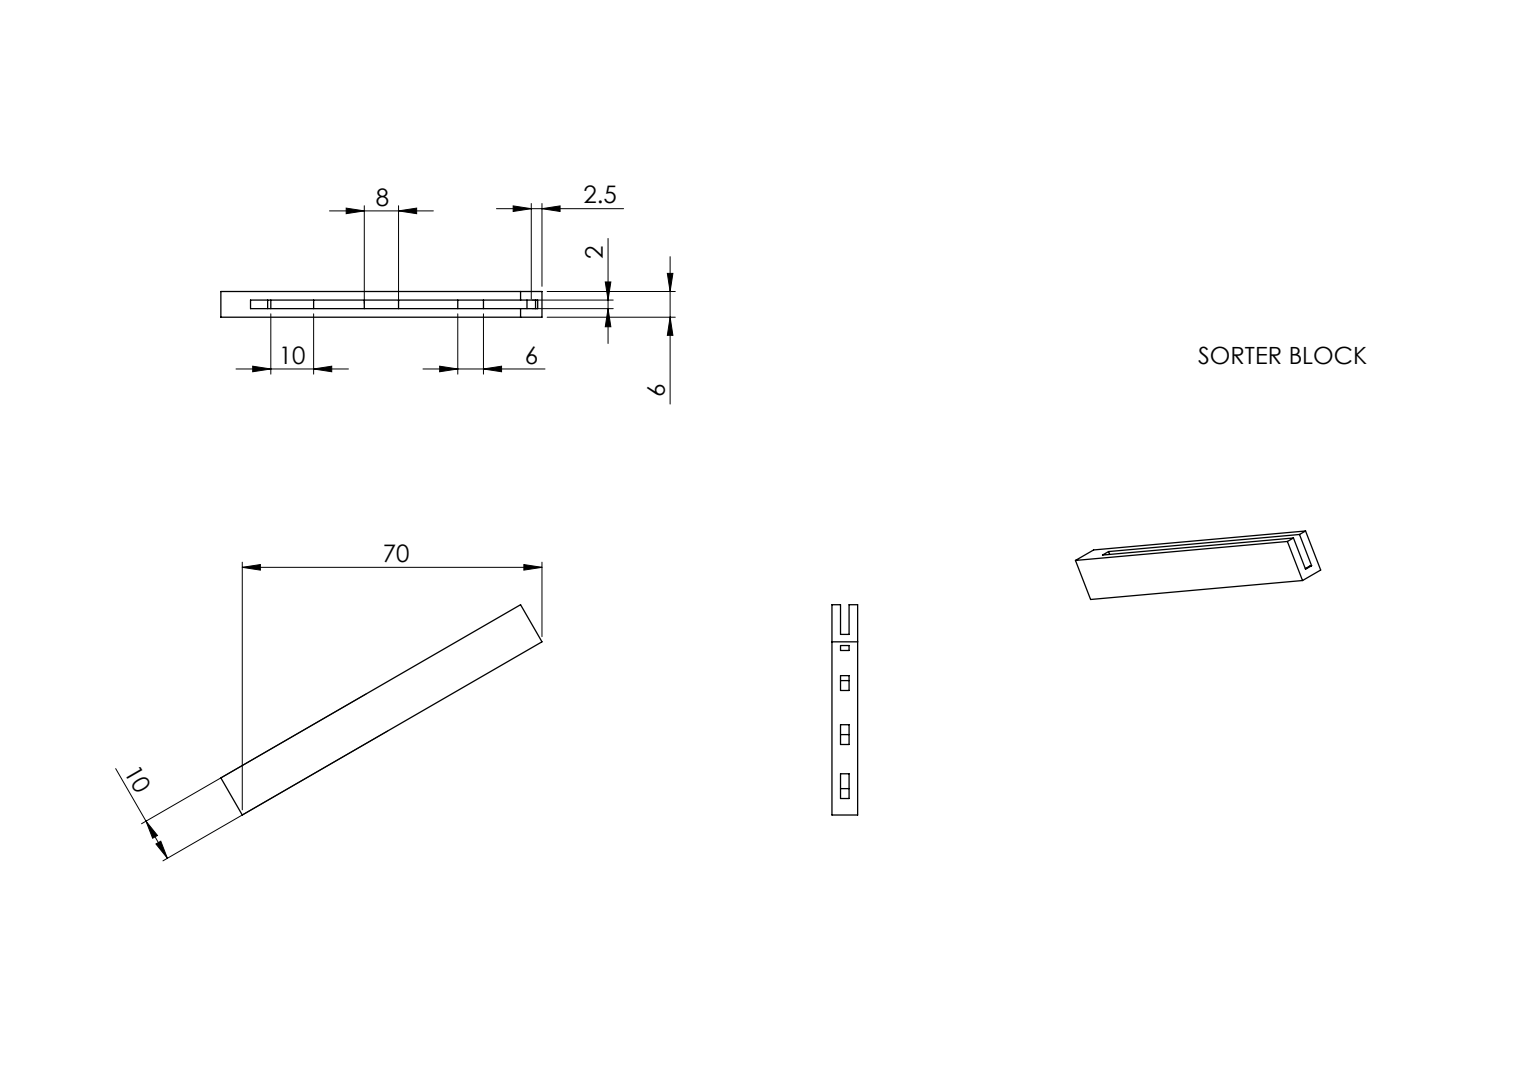
ISO-10303-21;
HEADER;
FILE_DESCRIPTION (('STEP AP214'),
    '1' );
FILE_NAME ('sorter block.step',
    '2026-10-26T05:17:54',
    ( '' ),
    ( '' ),
    'SwSTEP 2.0',
    'SolidWorks 2026',
    '' );
FILE_SCHEMA (( 'AUTOMOTIVE_DESIGN' ));
ENDSEC;

DATA;
#41=VERTEX_POINT ( 'NONE', #12875 ) ;
#78=PLANE ( 'NONE',  #12219 ) ;
#80=FACE_BOUND ( 'NONE', #12190, .T. ) ;
#96=FACE_OUTER_BOUND ( 'NONE', #3585, .T. ) ;
#117=CARTESIAN_POINT ( 'NONE',  ( -43.33333333333332860, 79.07477288111861924, -1.000000000000001110 ) ) ;
#136=EDGE_CURVE ( 'NONE', #12578, #3097, #7900, .T. ) ;
#159=LINE ( 'NONE', #2018, #4188 ) ;
#160=ORIENTED_EDGE ( 'NONE', *, *, #4406, .F. ) ;
#164=ORIENTED_EDGE ( 'NONE', *, *, #8938, .T. ) ;
#180=CARTESIAN_POINT ( 'NONE',  ( -56.80384757729341771, 34.46410161513777837, 0.000000000000000000 ) ) ;
#182=CARTESIAN_POINT ( 'NONE',  ( -60.38397459621558738, 30.66506350946110260, 0.000000000000000000 ) ) ;
#184=EDGE_CURVE ( 'NONE', #4807, #7972, #8814, .T. ) ;
#195=FACE_OUTER_BOUND ( 'NONE', #1919, .T. ) ;
#202=DIRECTION ( 'NONE',  ( -0.5000000000000042188, 0.8660254037844362651, 0.000000000000000000 ) ) ;
#240=ORIENTED_EDGE ( 'NONE', *, *, #10021, .T. ) ;
#255=VERTEX_POINT ( 'NONE', #12080 ) ;
#258=( GEOMETRIC_REPRESENTATION_CONTEXT ( 3 ) GLOBAL_UNCERTAINTY_ASSIGNED_CONTEXT ( ( #6606 ) ) GLOBAL_UNIT_ASSIGNED_CONTEXT ( ( #8219, #3259, #10305 ) ) REPRESENTATION_CONTEXT ( 'NONE', 'WORKASPACE' ) );
#263=AXIS2_PLACEMENT_3D ( 'NONE', #117, #3851, #2872 ) ;
#269=FACE_OUTER_BOUND ( 'NONE', #11895, .T. ) ;
#271=EDGE_CURVE ( 'NONE', #3833, #3097, #6317, .T. ) ;
#306=VECTOR ( 'NONE', #308, 1000.000000000000114 ) ;
#308=DIRECTION ( 'NONE',  ( 0.8660254037844361541, 0.5000000000000042188, 0.000000000000000000 ) ) ;
#315=ORIENTED_EDGE ( 'NONE', *, *, #7224, .T. ) ;
#329=DIRECTION ( 'NONE',  ( -0.8660254037844360431, -0.5000000000000045519, 0.000000000000000000 ) ) ;
#367=VECTOR ( 'NONE', #8627, 1000.000000000000114 ) ;
#377=CYLINDRICAL_SURFACE ( 'NONE', #4983, 1.500000000000000222 ) ;
#384=AXIS2_PLACEMENT_3D ( 'NONE', #10742, #1980, #7866 ) ;
#388=EDGE_CURVE ( 'NONE', #12930, #2334, #4689, .T. ) ;
#405=CARTESIAN_POINT ( 'NONE',  ( 37.99038105676688559, 21.93375672974103452, 1.000000000000000000 ) ) ;
#418=ORIENTED_EDGE ( 'NONE', *, *, #1473, .F. ) ;
#443=VERTEX_POINT ( 'NONE', #483 ) ;
#474=DIRECTION ( 'NONE',  ( -0.8660254037844360431, -0.5000000000000047740, -0.000000000000000000 ) ) ;
#477=CARTESIAN_POINT ( 'NONE',  ( -28.99038105676692112, 50.21281292110204930, -1.000000000000000000 ) ) ;
#481=CARTESIAN_POINT ( 'NONE',  ( 8.999999999999989342, 72.14656965084313356, -1.000000000000000000 ) ) ;
#483=CARTESIAN_POINT ( 'NONE',  ( 4.999999999999962697, 79.07477288111861924, 3.000000000000000000 ) ) ;
#484=ORIENTED_EDGE ( 'NONE', *, *, #7097, .F. ) ;
#486=DIRECTION ( 'NONE',  ( 4.336808689942017243E-16, 2.503857664561960972E-16, -1.000000000000000000 ) ) ;
#492=ORIENTED_EDGE ( 'NONE', *, *, #5266, .F. ) ;
#500=EDGE_CURVE ( 'NONE', #6408, #3143, #4030, .T. ) ;
#501=ORIENTED_EDGE ( 'NONE', *, *, #9357, .T. ) ;
#526=ORIENTED_EDGE ( 'NONE', *, *, #10407, .T. ) ;
#541=DIRECTION ( 'NONE',  ( 0.000000000000000000, 0.000000000000000000, 1.000000000000000000 ) ) ;
#568=ORIENTED_EDGE ( 'NONE', *, *, #10862, .T. ) ;
#570=CARTESIAN_POINT ( 'NONE',  ( 8.499999999999998224, 79.07477288111861924, 1.000000000000000000 ) ) ;
#576=ORIENTED_EDGE ( 'NONE', *, *, #12211, .T. ) ;
#606=FACE_OUTER_BOUND ( 'NONE', #6514, .T. ) ;
#625=DIRECTION ( 'NONE',  ( -0.8746197064978278313, 0.4848096214037562746, 1.049727191973305270E-16 ) ) ;
#645=VECTOR ( 'NONE', #10208, 1000.000000000000227 ) ;
#667=CARTESIAN_POINT ( 'NONE',  ( -54.07179676972453564, 35.73205080756890339, -1.000000000000000000 ) ) ;
#671=DIRECTION ( 'NONE',  ( 0.8660254037844361541, 0.5000000000000042188, 0.000000000000000000 ) ) ;
#676=ORIENTED_EDGE ( 'NONE', *, *, #11289, .T. ) ;
#685=DIRECTION ( 'NONE',  ( -0.8660254037844361541, -0.5000000000000042188, 9.389466242107218061E-17 ) ) ;
#690=VECTOR ( 'NONE', #8750, 1000.000000000000114 ) ;
#695=LINE ( 'NONE', #11320, #4590 ) ;
#724=ORIENTED_EDGE ( 'NONE', *, *, #4951, .F. ) ;
#728=DIRECTION ( 'NONE',  ( 0.000000000000000000, -1.000000000000000000, 0.000000000000000000 ) ) ;
#778=VECTOR ( 'NONE', #11676, 1000.000000000000000 ) ;
#803=CIRCLE ( 'NONE', #8129, 1.500000000000003331 ) ;
#820=PLANE ( 'NONE',  #10704 ) ;
#878=ORIENTED_EDGE ( 'NONE', *, *, #10870, .F. ) ;
#896=ORIENTED_EDGE ( 'NONE', *, *, #10776, .T. ) ;
#902=PLANE ( 'NONE',  #6579 ) ;
#922=LINE ( 'NONE', #11728, #1022 ) ;
#939=VECTOR ( 'NONE', #10169, 1000.000000000000000 ) ;
#943=DIRECTION ( 'NONE',  ( -0.000000000000000000, 0.000000000000000000, -1.000000000000000000 ) ) ;
#951=DIRECTION ( 'NONE',  ( 1.301042606982605124E-15, 7.511572993685881931E-16, 1.000000000000000000 ) ) ;
#1003=CARTESIAN_POINT ( 'NONE',  ( -43.33333333333332860, 79.07477288111861924, 0.9999999999999997780 ) ) ;
#1009=ORIENTED_EDGE ( 'NONE', *, *, #10776, .F. ) ;
#1022=VECTOR ( 'NONE', #6753, 1000.000000000000000 ) ;
#1031=FACE_OUTER_BOUND ( 'NONE', #3643, .T. ) ;
#1054=DIRECTION ( 'NONE',  ( 0.000000000000000000, 0.000000000000000000, -1.000000000000000000 ) ) ;
#1071=LINE ( 'NONE', #9053, #7641 ) ;
#1079=CARTESIAN_POINT ( 'NONE',  ( -58.07179676972458537, 42.66025403784442460, -1.000000000000000000 ) ) ;
#1092=ADVANCED_FACE ( 'NONE', ( #4448 ), #7017, .F. ) ;
#1115=PRODUCT_DEFINITION_FORMATION_WITH_SPECIFIED_SOURCE ( 'ANY', '', #8459, .NOT_KNOWN. ) ;
#1135=FACE_OUTER_BOUND ( 'NONE', #11908, .T. ) ;
#1138=LINE ( 'NONE', #9124, #5567 ) ;
#1144=DIRECTION ( 'NONE',  ( -0.8660254037844360431, -0.5000000000000047740, -0.000000000000000000 ) ) ;
#1156=DIRECTION ( 'NONE',  ( 0.000000000000000000, 0.000000000000000000, 1.000000000000000000 ) ) ;
#1161=ORIENTED_EDGE ( 'NONE', *, *, #4184, .T. ) ;
#1177=LINE ( 'NONE', #6217, #1912 ) ;
#1182=VECTOR ( 'NONE', #5508, 1000.000000000000114 ) ;
#1213=FILL_AREA_STYLE_COLOUR ( '', #7165 ) ;
#1245=LINE ( 'NONE', #182, #645 ) ;
#1282=DIRECTION ( 'NONE',  ( 0.8660254037844365982, 0.5000000000000036637, -0.000000000000000000 ) ) ;
#1292=VERTEX_POINT ( 'NONE', #10596 ) ;
#1293=EDGE_CURVE ( 'NONE', #4584, #1989, #12495, .T. ) ;
#1323=DIRECTION ( 'NONE',  ( 0.000000000000000000, -1.000000000000000000, 0.000000000000000000 ) ) ;
#1328=LINE ( 'NONE', #12388, #3779 ) ;
#1337=ORIENTED_EDGE ( 'NONE', *, *, #10803, .F. ) ;
#1352=CARTESIAN_POINT ( 'NONE',  ( -58.07179676972457116, 42.66025403784438907, 1.000000000000000000 ) ) ;
#1358=ORIENTED_EDGE ( 'NONE', *, *, #6254, .F. ) ;
#1361=EDGE_CURVE ( 'NONE', #7045, #2314, #5869, .T. ) ;
#1383=CARTESIAN_POINT ( 'NONE',  ( -9.666666666666658969, 61.36936462597000741, 0.9999999999999997780 ) ) ;
#1401=DIRECTION ( 'NONE',  ( -0.8660254037844361541, -0.5000000000000042188, 0.000000000000000000 ) ) ;
#1406=ORIENTED_EDGE ( 'NONE', *, *, #6522, .T. ) ;
#1423=CONICAL_SURFACE ( 'NONE', #8325, 1.500000000000003331, 1.029744259999999967 ) ;
#1434=DIRECTION ( 'NONE',  ( -0.8660254037844360431, -0.5000000000000047740, -0.000000000000000000 ) ) ;
#1452=ORIENTED_EDGE ( 'NONE', *, *, #2772, .T. ) ;
#1466=ADVANCED_FACE ( 'NONE', ( #96 ), #3984, .F. ) ;
#1473=EDGE_CURVE ( 'NONE', #443, #9678, #5994, .T. ) ;
#1478=VECTOR ( 'NONE', #7745, 1000.000000000000000 ) ;
#1480=LINE ( 'NONE', #2599, #10559 ) ;
#1482=VERTEX_POINT ( 'NONE', #4110 ) ;
#1484=CARTESIAN_POINT ( 'NONE',  ( -53.33333333333332149, 33.84900179459755520, 1.000000000000000888 ) ) ;
#1516=VERTEX_POINT ( 'NONE', #5340 ) ;
#1525=LINE ( 'NONE', #2520, #1780 ) ;
#1531=CARTESIAN_POINT ( 'NONE',  ( -31.49999999999998579, 46.45448267190452896, 3.000000000000000000 ) ) ;
#1534=LINE ( 'NONE', #7429, #778 ) ;
#1543=DIRECTION ( 'NONE',  ( 0.000000000000000000, 0.000000000000000000, 1.000000000000000000 ) ) ;
#1551=VECTOR ( 'NONE', #10036, 1000.000000000000000 ) ;
#1559=EDGE_CURVE ( 'NONE', #3514, #9678, #4177, .T. ) ;
#1587=LINE ( 'NONE', #7477, #8707 ) ;
#1602=DIRECTION ( 'NONE',  ( 0.000000000000000000, 0.000000000000000000, -1.000000000000000000 ) ) ;
#1617=LINE ( 'NONE', #1808, #7739 ) ;
#1648=ORIENTED_EDGE ( 'NONE', *, *, #1559, .T. ) ;
#1663=VECTOR ( 'NONE', #5897, 1000.000000000000000 ) ;
#1675=EDGE_CURVE ( 'NONE', #7045, #4305, #3650, .T. ) ;
#1711=ORIENTED_EDGE ( 'NONE', *, *, #12047, .T. ) ;
#1738=EDGE_CURVE ( 'NONE', #4892, #12446, #1480, .T. ) ;
#1742=LINE ( 'NONE', #5730, #2308 ) ;
#1755=VECTOR ( 'NONE', #9529, 1000.000000000000000 ) ;
#1766=EDGE_CURVE ( 'NONE', #8153, #11802, #9655, .T. ) ;
#1780=VECTOR ( 'NONE', #5516, 1000.000000000000227 ) ;
#1799=EDGE_CURVE ( 'NONE', #4047, #2314, #7503, .T. ) ;
#1808=CARTESIAN_POINT ( 'NONE',  ( -28.99038105676692112, 50.21281292110204930, -1.000000000000000000 ) ) ;
#1809=DIRECTION ( 'NONE',  ( 1.000000000000000000, 0.000000000000000000, -0.000000000000000000 ) ) ;
#1819=DIRECTION ( 'NONE',  ( 0.8660254037844361541, 0.5000000000000042188, 0.000000000000000000 ) ) ;
#1829=DIRECTION ( 'NONE',  ( -0.5000000000000043299, 0.8660254037844362651, 0.000000000000000000 ) ) ;
#1885=ORIENTED_EDGE ( 'NONE', *, *, #2003, .F. ) ;
#1912=VECTOR ( 'NONE', #5237, 1000.000000000000114 ) ;
#1917=CARTESIAN_POINT ( 'NONE',  ( -43.33333333333332860, 39.62250448649387380, 3.000000000000000000 ) ) ;
#1919=EDGE_LOOP ( 'NONE', ( #1358, #1009, #9756, #4335 ) ) ;
#1922=MECHANICAL_DESIGN_GEOMETRIC_PRESENTATION_REPRESENTATION('',(#11529),#10056);
#1923=CARTESIAN_POINT ( 'NONE',  ( 37.99038105676688559, 21.93375672974103452, -1.000000000000000000 ) ) ;
#1948=CARTESIAN_POINT ( 'NONE',  ( 4.999999999999962697, 79.07477288111861924, 3.000000000000000000 ) ) ;
#1962=EDGE_CURVE ( 'NONE', #3599, #4788, #1071, .T. ) ;
#1980=DIRECTION ( 'NONE',  ( -0.5000000000000043299, 0.8660254037844362651, 0.000000000000000000 ) ) ;
#1989=VERTEX_POINT ( 'NONE', #3970 ) ;
#2003=EDGE_CURVE ( 'NONE', #2627, #1292, #4292, .T. ) ;
#2015=ORIENTED_EDGE ( 'NONE', *, *, #5500, .T. ) ;
#2018=CARTESIAN_POINT ( 'NONE',  ( -65.00000000000004263, 38.66025403784436065, -3.000000000000000000 ) ) ;
#2040=ADVANCED_FACE ( 'NONE', ( #11080, #2132, #1135, #10367, #80 ), #4099, .F. ) ;
#2046=ORIENTED_EDGE ( 'NONE', *, *, #7362, .F. ) ;
#2059=FACE_OUTER_BOUND ( 'NONE', #3684, .T. ) ;
#2089=CARTESIAN_POINT ( 'NONE',  ( -31.49999999999998579, 46.45448267190452896, 1.000000000000000000 ) ) ;
#2118=PLANE ( 'NONE',  #3215 ) ;
#2132=FACE_BOUND ( 'NONE', #11150, .T. ) ;
#2138=( LENGTH_UNIT ( ) NAMED_UNIT ( * ) SI_UNIT ( .MILLI., .METRE. ) );
#2163=ORIENTED_EDGE ( 'NONE', *, *, #10289, .T. ) ;
#2168=ADVANCED_FACE ( 'NONE', ( #606 ), #12528, .T. ) ;
#2180=ORIENTED_EDGE ( 'NONE', *, *, #1766, .F. ) ;
#2181=CARTESIAN_POINT ( 'NONE',  ( -23.49999999999999289, 79.07477288111861924, 1.000000000000000000 ) ) ;
#2192=PLANE ( 'NONE',  #10824 ) ;
#2205=ORIENTED_EDGE ( 'NONE', *, *, #7737, .T. ) ;
#2216=ORIENTED_EDGE ( 'NONE', *, *, #3696, .T. ) ;
#2229=CARTESIAN_POINT ( 'NONE',  ( -61.00000000000000711, 31.73205080756887142, 3.000000000000000000 ) ) ;
#2239=CARTESIAN_POINT ( 'NONE',  ( -61.13397459621560159, 31.96410161513775350, 0.000000000000000000 ) ) ;
#2255=ORIENTED_EDGE ( 'NONE', *, *, #9162, .T. ) ;
#2298=ORIENTED_EDGE ( 'NONE', *, *, #11289, .F. ) ;
#2308=VECTOR ( 'NONE', #625, 1000.000000000000114 ) ;
#2314=VERTEX_POINT ( 'NONE', #4479 ) ;
#2334=VERTEX_POINT ( 'NONE', #3956 ) ;
#2347=VERTEX_POINT ( 'NONE', #8789 ) ;
#2357=PLANE ( 'NONE',  #4716 ) ;
#2372=ORIENTED_EDGE ( 'NONE', *, *, #10388, .F. ) ;
#2412=EDGE_LOOP ( 'NONE', ( #6661, #9476, #10070 ) ) ;
#2435=ORIENTED_EDGE ( 'NONE', *, *, #4012, .T. ) ;
#2479=CARTESIAN_POINT ( 'NONE',  ( -60.00000000000000000, 30.00000000000000000, -1.000000000000000000 ) ) ;
#2495=ORIENTED_EDGE ( 'NONE', *, *, #1293, .F. ) ;
#2497=ORIENTED_EDGE ( 'NONE', *, *, #1962, .T. ) ;
#2498=ADVANCED_FACE ( 'NONE', ( #3366, #195 ), #2118, .T. ) ;
#2520=CARTESIAN_POINT ( 'NONE',  ( -53.07079676972452376, 33.99826794919245998, -1.000000000000000000 ) ) ;
#2537=ORIENTED_EDGE ( 'NONE', *, *, #6254, .T. ) ;
#2538=DIRECTION ( 'NONE',  ( -0.8660254037844359321, -0.5000000000000046629, -0.000000000000000000 ) ) ;
#2541=CARTESIAN_POINT ( 'NONE',  ( -53.33333333333332149, 36.15840287135605990, 1.000000000000000888 ) ) ;
#2553=DIRECTION ( 'NONE',  ( -0.5000000000000045519, 0.8660254037844360431, 0.000000000000000000 ) ) ;
#2564=ORIENTED_EDGE ( 'NONE', *, *, #10426, .F. ) ;
#2578=CARTESIAN_POINT ( 'NONE',  ( -65.00000000000004263, 38.66025403784436065, 3.000000000000000000 ) ) ;
#2594=CARTESIAN_POINT ( 'NONE',  ( -31.49999999999998579, 48.76388374866304076, 1.000000000000000000 ) ) ;
#2599=CARTESIAN_POINT ( 'NONE',  ( -61.88397459621560870, 33.26313972081441506, 1.836970198721030427E-16 ) ) ;
#2602=DIRECTION ( 'NONE',  ( 0.5000000000000049960, -0.8660254037844357100, 0.000000000000000000 ) ) ;
#2617=ORIENTED_EDGE ( 'NONE', *, *, #10476, .F. ) ;
#2619=PRODUCT_CONTEXT ( 'NONE', #12365, 'mechanical' ) ;
#2627=VERTEX_POINT ( 'NONE', #6486 ) ;
#2628=VECTOR ( 'NONE', #10063, 1000.000000000000000 ) ;
#2630=LINE ( 'NONE', #3357, #2896 ) ;
#2633=ORIENTED_EDGE ( 'NONE', *, *, #1361, .T. ) ;
#2642=DIRECTION ( 'NONE',  ( -0.8660254037844360431, -0.5000000000000047740, -0.000000000000000000 ) ) ;
#2654=DIRECTION ( 'NONE',  ( 0.8660254037844361541, 0.5000000000000045519, -0.000000000000000000 ) ) ;
#2755=ORIENTED_EDGE ( 'NONE', *, *, #4012, .F. ) ;
#2766=ADVANCED_FACE ( 'NONE', ( #9221 ), #3016, .T. ) ;
#2772=EDGE_CURVE ( 'NONE', #8971, #3649, #7767, .T. ) ;
#2856=EDGE_CURVE ( 'NONE', #10254, #10113, #6847, .T. ) ;
#2867=ORIENTED_EDGE ( 'NONE', *, *, #8911, .F. ) ;
#2869=DIRECTION ( 'NONE',  ( 4.336808689942017243E-16, 0.000000000000000000, -1.000000000000000000 ) ) ;
#2872=DIRECTION ( 'NONE',  ( 0.000000000000000000, 0.000000000000000000, 1.000000000000000000 ) ) ;
#2896=VECTOR ( 'NONE', #5363, 1000.000000000000000 ) ;
#2918=DIRECTION ( 'NONE',  ( -0.8660254037844361541, -0.5000000000000042188, 0.000000000000000000 ) ) ;
#2937=EDGE_LOOP ( 'NONE', ( #5814, #4900, #5525, #676 ) ) ;
#2998=ADVANCED_FACE ( 'NONE', ( #4238 ), #12013, .T. ) ;
#3002=VECTOR ( 'NONE', #951, 1000.000000000000000 ) ;
#3003=ORIENTED_EDGE ( 'NONE', *, *, #6590, .F. ) ;
#3016=PLANE ( 'NONE',  #263 ) ;
#3050=AXIS2_PLACEMENT_3D ( 'NONE', #12331, #8279, #1401 ) ;
#3064=EDGE_LOOP ( 'NONE', ( #2298, #2564 ) ) ;
#3074=CARTESIAN_POINT ( 'NONE',  ( -61.00000000000000711, 31.73205080756887142, 3.000000000000000000 ) ) ;
#3097=VERTEX_POINT ( 'NONE', #481 ) ;
#3105=LINE ( 'NONE', #1923, #3786 ) ;
#3123=SURFACE_STYLE_FILL_AREA ( #4362 ) ;
#3131=ORIENTED_EDGE ( 'NONE', *, *, #9805, .F. ) ;
#3134=ORIENTED_EDGE ( 'NONE', *, *, #4074, .T. ) ;
#3135=VECTOR ( 'NONE', #4800, 1000.000000000000000 ) ;
#3143=VERTEX_POINT ( 'NONE', #3820 ) ;
#3185=CARTESIAN_POINT ( 'NONE',  ( 6.500000000000000000, 79.07477288111861924, -1.000000000000000222 ) ) ;
#3188=CARTESIAN_POINT ( 'NONE',  ( -61.00000000000000711, 31.73205080756887142, 3.000000000000000000 ) ) ;
#3196=ORIENTED_EDGE ( 'NONE', *, *, #10476, .T. ) ;
#3204=VERTEX_POINT ( 'NONE', #3517 ) ;
#3207=CARTESIAN_POINT ( 'NONE',  ( 0.000000000000000000, 0.000000000000000000, 3.000000000000000000 ) ) ;
#3215=AXIS2_PLACEMENT_3D ( 'NONE', #3235, #329, #4083 ) ;
#3219=DIRECTION ( 'NONE',  ( -0.8660254037844360431, -0.5000000000000047740, -0.000000000000000000 ) ) ;
#3235=CARTESIAN_POINT ( 'NONE',  ( -60.00000000000000000, 30.00000000000000000, 3.000000000000000000 ) ) ;
#3259=( NAMED_UNIT ( * ) PLANE_ANGLE_UNIT ( ) SI_UNIT ( $, .RADIAN. ) );
#3260=EDGE_CURVE ( 'NONE', #41, #3601, #8442, .T. ) ;
#3267=ORIENTED_EDGE ( 'NONE', *, *, #7224, .F. ) ;
#3270=ORIENTED_EDGE ( 'NONE', *, *, #11837, .T. ) ;
#3304=AXIS2_PLACEMENT_3D ( 'NONE', #3188, #12206, #7237 ) ;
#3326=UNCERTAINTY_MEASURE_WITH_UNIT (LENGTH_MEASURE( 1.000000000000000082E-05 ), #11835, 'distance_accuracy_value', 'NONE');
#3337=VECTOR ( 'NONE', #7159, 1000.000000000000114 ) ;
#3357=CARTESIAN_POINT ( 'NONE',  ( -53.33333333333332149, 33.84900179459754810, 3.000000000000000000 ) ) ;
#3366=FACE_BOUND ( 'NONE', #3064, .T. ) ;
#3377=DIRECTION ( 'NONE',  ( 8.673617379884034486E-16, 0.000000000000000000, -1.000000000000000000 ) ) ;
#3419=VERTEX_POINT ( 'NONE', #12351 ) ;
#3425=ORIENTED_EDGE ( 'NONE', *, *, #11602, .T. ) ;
#3442=EDGE_CURVE ( 'NONE', #12578, #2627, #4371, .T. ) ;
#3455=EDGE_LOOP ( 'NONE', ( #10721, #12724, #9171, #8954 ) ) ;
#3478=DIRECTION ( 'NONE',  ( 0.8660254037844361541, 0.5000000000000042188, 0.000000000000000000 ) ) ;
#3498=AXIS2_PLACEMENT_3D ( 'NONE', #12393, #474, #5590 ) ;
#3513=DIRECTION ( 'NONE',  ( 0.8660254037844361541, 0.5000000000000042188, 0.000000000000000000 ) ) ;
#3514=VERTEX_POINT ( 'NONE', #1352 ) ;
#3517=CARTESIAN_POINT ( 'NONE',  ( -56.02330673931587768, 34.91474707805760858, 0.000000000000000000 ) ) ;
#3523=VECTOR ( 'NONE', #11007, 1000.000000000000114 ) ;
#3525=DIRECTION ( 'NONE',  ( 0.000000000000000000, -1.000000000000000000, 0.000000000000000000 ) ) ;
#3538=CARTESIAN_POINT ( 'NONE',  ( -60.00000000000000000, 30.00000000000000000, 3.000000000000000000 ) ) ;
#3577=CARTESIAN_POINT ( 'NONE',  ( -57.55384757729342482, 35.76313972081443637, 1.836970198721030427E-16 ) ) ;
#3585=EDGE_LOOP ( 'NONE', ( #3003, #11479, #10078, #8240 ) ) ;
#3593=ORIENTED_EDGE ( 'NONE', *, *, #7780, .F. ) ;
#3599=VERTEX_POINT ( 'NONE', #11425 ) ;
#3601=VERTEX_POINT ( 'NONE', #2541 ) ;
#3621=ORIENTED_EDGE ( 'NONE', *, *, #8569, .F. ) ;
#3629=EDGE_CURVE ( 'NONE', #9137, #9525, #4696, .T. ) ;
#3639=ORIENTED_EDGE ( 'NONE', *, *, #1361, .F. ) ;
#3643=EDGE_LOOP ( 'NONE', ( #6511, #7441, #4312, #2495 ) ) ;
#3649=VERTEX_POINT ( 'NONE', #1484 ) ;
#3650=LINE ( 'NONE', #10580, #6575 ) ;
#3684=EDGE_LOOP ( 'NONE', ( #4513, #2497, #526, #11444, #4882, #8285, #9279, #10500 ) ) ;
#3696=EDGE_CURVE ( 'NONE', #9525, #4047, #3715, .T. ) ;
#3715=LINE ( 'NONE', #7699, #10578 ) ;
#3717=VECTOR ( 'NONE', #3513, 1000.000000000000114 ) ;
#3763=LINE ( 'NONE', #7553, #4411 ) ;
#3766=ADVANCED_FACE ( 'NONE', ( #9913 ), #3841, .T. ) ;
#3773=PLANE ( 'NONE',  #10329 ) ;
#3777=VECTOR ( 'NONE', #6628, 1000.000000000000000 ) ;
#3778=LINE ( 'NONE', #11748, #6485 ) ;
#3779=VECTOR ( 'NONE', #4224, 1000.000000000000114 ) ;
#3786=VECTOR ( 'NONE', #5903, 1000.000000000000000 ) ;
#3799=EDGE_CURVE ( 'NONE', #10113, #6517, #12073, .T. ) ;
#3800=CARTESIAN_POINT ( 'NONE',  ( 6.499999999999999112, 70.70319397786906279, 3.000000000000039080 ) ) ;
#3820=CARTESIAN_POINT ( 'NONE',  ( -31.49999999999998579, 46.45448267190452185, -1.000000000000000000 ) ) ;
#3832=CARTESIAN_POINT ( 'NONE',  ( -9.666666666666657193, 59.05996354921150271, 1.000000000000000000 ) ) ;
#3833=VERTEX_POINT ( 'NONE', #8282 ) ;
#3837=EDGE_CURVE ( 'NONE', #4305, #7601, #1138, .T. ) ;
#3841=PLANE ( 'NONE',  #12680 ) ;
#3851=DIRECTION ( 'NONE',  ( -1.000000000000000000, 0.000000000000000000, 0.000000000000000000 ) ) ;
#3886=FACE_OUTER_BOUND ( 'NONE', #9493, .T. ) ;
#3893=ORIENTED_EDGE ( 'NONE', *, *, #11837, .F. ) ;
#3928=( NAMED_UNIT ( * ) SI_UNIT ( $, .STERADIAN. ) SOLID_ANGLE_UNIT ( ) );
#3937=ORIENTED_EDGE ( 'NONE', *, *, #1799, .F. ) ;
#3939=ORIENTED_EDGE ( 'NONE', *, *, #12047, .F. ) ;
#3956=CARTESIAN_POINT ( 'NONE',  ( 9.999999999999994671, 70.41451884327426569, -3.000000000000000000 ) ) ;
#3970=CARTESIAN_POINT ( 'NONE',  ( -65.00000000000004263, 38.66025403784436065, 3.000000000000000000 ) ) ;
#3977=ADVANCED_FACE ( 'NONE', ( #8410 ), #6821, .F. ) ;
#3980=CARTESIAN_POINT ( 'NONE',  ( -60.00000000000000000, 30.00000000000000000, 1.000000000000001776 ) ) ;
#3984=CYLINDRICAL_SURFACE ( 'NONE', #6794, 1.500000000000000222 ) ;
#3992=EDGE_CURVE ( 'NONE', #11985, #3143, #10495, .T. ) ;
#4012=EDGE_CURVE ( 'NONE', #8585, #6517, #10433, .T. ) ;
#4030=LINE ( 'NONE', #9906, #10326 ) ;
#4032=CARTESIAN_POINT ( 'NONE',  ( 6.499999999999999112, 79.07477288111861924, 0.9999999999999997780 ) ) ;
#4043=MECHANICAL_DESIGN_GEOMETRIC_PRESENTATION_REPRESENTATION('',(#8836),#11760);
#4047=VERTEX_POINT ( 'NONE', #5053 ) ;
#4068=LINE ( 'NONE', #7860, #7552 ) ;
#4074=EDGE_CURVE ( 'NONE', #2347, #11985, #7410, .T. ) ;
#4083=DIRECTION ( 'NONE',  ( 0.5000000000000045519, -0.8660254037844360431, 0.000000000000000000 ) ) ;
#4095=CARTESIAN_POINT ( 'NONE',  ( 0.000000000000000000, 0.000000000000000000, -3.000000000000000000 ) ) ;
#4098=AXIS2_PLACEMENT_3D ( 'NONE', #9382, #2654, #11473 ) ;
#4099=PLANE ( 'NONE',  #3050 ) ;
#4110=CARTESIAN_POINT ( 'NONE',  ( 4.999999999999962697, 79.07477288111861924, -3.000000000000000000 ) ) ;
#4127=ORIENTED_EDGE ( 'NONE', *, *, #12932, .T. ) ;
#4132=DIRECTION ( 'NONE',  ( 0.5000000000000038858, -0.8660254037844362651, 0.000000000000000000 ) ) ;
#4144=CARTESIAN_POINT ( 'NONE',  ( 0.000000000000000000, 0.000000000000000000, -1.000000000000000000 ) ) ;
#4153=CARTESIAN_POINT ( 'NONE',  ( -60.00000000000000000, 30.00000000000000000, -3.000000000000000000 ) ) ;
#4157=DIRECTION ( 'NONE',  ( 0.000000000000000000, 0.000000000000000000, -1.000000000000000000 ) ) ;
#4167=CARTESIAN_POINT ( 'NONE',  ( 4.999999999999962697, 79.07477288111861924, -1.000000000000000000 ) ) ;
#4175=DIRECTION ( 'NONE',  ( 0.000000000000000000, 0.000000000000000000, -1.000000000000000000 ) ) ;
#4177=LINE ( 'NONE', #9268, #9301 ) ;
#4184=EDGE_CURVE ( 'NONE', #10254, #8585, #1587, .T. ) ;
#4188=VECTOR ( 'NONE', #12085, 1000.000000000000114 ) ;
#4224=DIRECTION ( 'NONE',  ( 0.8660254037844361541, 0.5000000000000042188, 0.000000000000000000 ) ) ;
#4238=FACE_OUTER_BOUND ( 'NONE', #4837, .T. ) ;
#4248=ORIENTED_EDGE ( 'NONE', *, *, #10870, .T. ) ;
#4250=FACE_OUTER_BOUND ( 'NONE', #7438, .T. ) ;
#4292=LINE ( 'NONE', #5385, #939 ) ;
#4305=VERTEX_POINT ( 'NONE', #4666 ) ;
#4312=ORIENTED_EDGE ( 'NONE', *, *, #6671, .F. ) ;
#4335=ORIENTED_EDGE ( 'NONE', *, *, #9302, .T. ) ;
#4346=CARTESIAN_POINT ( 'NONE',  ( -60.00000000000000000, 30.00000000000000000, -3.000000000000000000 ) ) ;
#4362=FILL_AREA_STYLE ('',( #1213 ) ) ;
#4371=LINE ( 'NONE', #10253, #12462 ) ;
#4374=VECTOR ( 'NONE', #9444, 1000.000000000000114 ) ;
#4382=CARTESIAN_POINT ( 'NONE',  ( -28.99038105676692112, 50.21281292110204930, 1.000000000000000000 ) ) ;
#4406=EDGE_CURVE ( 'NONE', #3143, #7972, #7701, .T. ) ;
#4411=VECTOR ( 'NONE', #541, 1000.000000000000000 ) ;
#4423=CARTESIAN_POINT ( 'NONE',  ( -23.49999999999999289, 53.38268590218009280, -1.000000000000000000 ) ) ;
#4448=FACE_OUTER_BOUND ( 'NONE', #12596, .T. ) ;
#4479=CARTESIAN_POINT ( 'NONE',  ( -43.33333333333332149, 39.62250448649387380, -1.000000000000000888 ) ) ;
#4488=AXIS2_PLACEMENT_3D ( 'NONE', #4144, #1054, #5418 ) ;
#4512=CARTESIAN_POINT ( 'NONE',  ( -3.666666666666663410, 62.52406516434930239, -1.000000000000000888 ) ) ;
#4513=ORIENTED_EDGE ( 'NONE', *, *, #7362, .T. ) ;
#4520=VECTOR ( 'NONE', #10450, 1000.000000000000114 ) ;
#4527=ORIENTED_EDGE ( 'NONE', *, *, #184, .T. ) ;
#4528=VECTOR ( 'NONE', #11282, 1000.000000000000000 ) ;
#4534=FACE_OUTER_BOUND ( 'NONE', #9426, .T. ) ;
#4584=VERTEX_POINT ( 'NONE', #12866 ) ;
#4590=VECTOR ( 'NONE', #6285, 1000.000000000000000 ) ;
#4616=DIRECTION ( 'NONE',  ( 1.301042606982605124E-15, 7.511572993685881931E-16, 1.000000000000000000 ) ) ;
#4627=DIRECTION ( 'NONE',  ( 0.8660254037844361541, 0.5000000000000042188, -9.389466242107221759E-17 ) ) ;
#4639=CARTESIAN_POINT ( 'NONE',  ( -60.00000000000000000, 30.00000000000000000, -0.9999999999999947820 ) ) ;
#4651=EDGE_CURVE ( 'NONE', #8770, #4892, #9964, .T. ) ;
#4666=CARTESIAN_POINT ( 'NONE',  ( -43.33333333333332860, 41.93190556325237850, 1.000000000000000000 ) ) ;
#4689=LINE ( 'NONE', #10577, #1755 ) ;
#4696=LINE ( 'NONE', #5608, #4520 ) ;
#4716=AXIS2_PLACEMENT_3D ( 'NONE', #5353, #9348, #8504 ) ;
#4720=CARTESIAN_POINT ( 'NONE',  ( -31.49999999999998579, 79.07477288111861924, -1.000000000000000000 ) ) ;
#4773=ORIENTED_EDGE ( 'NONE', *, *, #184, .F. ) ;
#4788=VERTEX_POINT ( 'NONE', #4167 ) ;
#4796=ADVANCED_FACE ( 'NONE', ( #11346 ), #12142, .T. ) ;
#4800=DIRECTION ( 'NONE',  ( 0.5000000000000036637, -0.8660254037844365982, 0.000000000000000000 ) ) ;
#4807=VERTEX_POINT ( 'NONE', #4423 ) ;
#4809=LINE ( 'NONE', #5908, #6840 ) ;
#4820=ORIENTED_EDGE ( 'NONE', *, *, #1675, .F. ) ;
#4824=DIRECTION ( 'NONE',  ( 0.000000000000000000, 0.000000000000000000, 1.000000000000000000 ) ) ;
#4827=CARTESIAN_POINT ( 'NONE',  ( -9.666666666666657193, 79.07477288111861924, -1.000000000000000000 ) ) ;
#4837=EDGE_LOOP ( 'NONE', ( #6312, #11593, #4902, #10218, #418, #7945, #10787, #6269 ) ) ;
#4858=EDGE_CURVE ( 'NONE', #7601, #6408, #1534, .T. ) ;
#4868=ORIENTED_EDGE ( 'NONE', *, *, #8542, .F. ) ;
#4882=ORIENTED_EDGE ( 'NONE', *, *, #9302, .F. ) ;
#4886=DIRECTION ( 'NONE',  ( 1.000000000000000000, 0.000000000000000000, 0.000000000000000000 ) ) ;
#4892=VERTEX_POINT ( 'NONE', #3577 ) ;
#4900=ORIENTED_EDGE ( 'NONE', *, *, #4651, .F. ) ;
#4902=ORIENTED_EDGE ( 'NONE', *, *, #271, .F. ) ;
#4908=DIRECTION ( 'NONE',  ( -0.000000000000000000, 0.000000000000000000, -1.000000000000000000 ) ) ;
#4949=CARTESIAN_POINT ( 'NONE',  ( 8.499999999999989342, 69.54849343948980334, -1.000000000000000000 ) ) ;
#4951=EDGE_CURVE ( 'NONE', #7045, #6408, #6568, .T. ) ;
#4966=ORIENTED_EDGE ( 'NONE', *, *, #4951, .T. ) ;
#4971=EDGE_CURVE ( 'NONE', #3204, #8770, #4809, .T. ) ;
#4973=EDGE_LOOP ( 'NONE', ( #8310, #3270, #3131, #6871 ) ) ;
#4982=CARTESIAN_POINT ( 'NONE',  ( -43.33333333333332860, 41.93190556325238560, -1.000000000000001110 ) ) ;
#4983=AXIS2_PLACEMENT_3D ( 'NONE', #2239, #1434, #8119 ) ;
#5017=ORIENTED_EDGE ( 'NONE', *, *, #3260, .F. ) ;
#5024=PLANE ( 'NONE',  #11944 ) ;
#5046=LINE ( 'NONE', #12718, #3135 ) ;
#5048=ORIENTED_EDGE ( 'NONE', *, *, #8911, .T. ) ;
#5053=CARTESIAN_POINT ( 'NONE',  ( -53.33333333333332149, 33.84900179459754810, -0.9999999999999997780 ) ) ;
#5066=VERTEX_POINT ( 'NONE', #3832 ) ;
#5077=CARTESIAN_POINT ( 'NONE',  ( -43.33333333333332860, 79.07477288111861924, -1.000000000000001110 ) ) ;
#5093=ORIENTED_EDGE ( 'NONE', *, *, #8064, .F. ) ;
#5127=DIRECTION ( 'NONE',  ( 0.000000000000000000, -1.000000000000000000, 0.000000000000000000 ) ) ;
#5154=PLANE ( 'NONE',  #12716 ) ;
#5159=LINE ( 'NONE', #4382, #306 ) ;
#5167=ORIENTED_EDGE ( 'NONE', *, *, #388, .F. ) ;
#5188=EDGE_CURVE ( 'NONE', #7039, #2334, #5319, .T. ) ;
#5194=ADVANCED_FACE ( 'NONE', ( #2059 ), #2192, .T. ) ;
#5200=CARTESIAN_POINT ( 'NONE',  ( -3.666666666666659413, 79.07477288111861924, 0.9999999999999991118 ) ) ;
#5214=ORIENTED_EDGE ( 'NONE', *, *, #9357, .F. ) ;
#5237=DIRECTION ( 'NONE',  ( -0.8660254037844361541, -0.5000000000000042188, -9.389466242107216828E-17 ) ) ;
#5244=ORIENTED_EDGE ( 'NONE', *, *, #3629, .T. ) ;
#5266=EDGE_CURVE ( 'NONE', #7601, #11985, #12453, .T. ) ;
#5290=PRODUCT_DEFINITION ( 'UNKNOWN', '', #1115, #9731 ) ;
#5318=CARTESIAN_POINT ( 'NONE',  ( -53.33333333333332149, 79.07477288111861924, 1.000000000000000888 ) ) ;
#5319=LINE ( 'NONE', #4153, #3523 ) ;
#5326=DIRECTION ( 'NONE',  ( 0.5000000000000036637, -0.8660254037844365982, 0.000000000000000000 ) ) ;
#5340=CARTESIAN_POINT ( 'NONE',  ( 6.499999999999999112, 70.70319397786906279, 0.9999999999999997780 ) ) ;
#5353=CARTESIAN_POINT ( 'NONE',  ( -23.49999999999999289, 79.07477288111861924, -1.000000000000000000 ) ) ;
#5354=VERTEX_POINT ( 'NONE', #11463 ) ;
#5363=DIRECTION ( 'NONE',  ( 0.000000000000000000, 0.000000000000000000, -1.000000000000000000 ) ) ;
#5385=CARTESIAN_POINT ( 'NONE',  ( 8.499999999999998224, 79.07477288111861924, 1.000000000000000000 ) ) ;
#5386=LINE ( 'NONE', #405, #5647 ) ;
#5389=ORIENTED_EDGE ( 'NONE', *, *, #7780, .T. ) ;
#5409=DIRECTION ( 'NONE',  ( 0.000000000000000000, 0.000000000000000000, -1.000000000000000000 ) ) ;
#5416=FACE_OUTER_BOUND ( 'NONE', #6675, .T. ) ;
#5418=DIRECTION ( 'NONE',  ( -1.000000000000000000, 0.000000000000000000, -0.000000000000000000 ) ) ;
#5500=EDGE_CURVE ( 'NONE', #3649, #4047, #2630, .T. ) ;
#5508=DIRECTION ( 'NONE',  ( -0.8660254037844361541, -0.5000000000000042188, 0.000000000000000000 ) ) ;
#5515=DIRECTION ( 'NONE',  ( 0.8660254037844362651, 0.5000000000000042188, 0.000000000000000000 ) ) ;
#5516=DIRECTION ( 'NONE',  ( -0.5000000000000044409, 0.8660254037844360431, 0.000000000000000000 ) ) ;
#5525=ORIENTED_EDGE ( 'NONE', *, *, #11663, .T. ) ;
#5540=ORIENTED_EDGE ( 'NONE', *, *, #7598, .T. ) ;
#5541=DIRECTION ( 'NONE',  ( 0.8660254037844361541, 0.5000000000000042188, 0.000000000000000000 ) ) ;
#5567=VECTOR ( 'NONE', #7235, 1000.000000000000114 ) ;
#5590=DIRECTION ( 'NONE',  ( 0.5000000000000038858, -0.8660254037844362651, 0.000000000000000000 ) ) ;
#5608=CARTESIAN_POINT ( 'NONE',  ( -28.99038105676692112, 50.21281292110204930, -1.000000000000000000 ) ) ;
#5615=LINE ( 'NONE', #4639, #367 ) ;
#5641=CARTESIAN_POINT ( 'NONE',  ( -3.666666666666661634, 79.07477288111861924, -1.000000000000000666 ) ) ;
#5647=VECTOR ( 'NONE', #5326, 1000.000000000000000 ) ;
#5664=ORIENTED_EDGE ( 'NONE', *, *, #271, .T. ) ;
#5670=ORIENTED_EDGE ( 'NONE', *, *, #3992, .T. ) ;
#5704=AXIS2_PLACEMENT_3D ( 'NONE', #8997, #4824, #4886 ) ;
#5713=CARTESIAN_POINT ( 'NONE',  ( -60.00000000000000000, 30.00000000000000000, -1.000000000000000000 ) ) ;
#5717=LINE ( 'NONE', #9580, #1478 ) ;
#5730=CARTESIAN_POINT ( 'NONE',  ( -57.55384757729342482, 35.76313972081443637, 1.836970198721030427E-16 ) ) ;
#5759=EDGE_LOOP ( 'NONE', ( #5017, #4127, #1648, #12677, #10198, #6739, #3425, #11611, #9417, #12912, #6780, #10968, #3621, #501, #3134, #492, #6263, #5389, #1452, #3939 ) ) ;
#5790=FACE_OUTER_BOUND ( 'NONE', #8700, .T. ) ;
#5794=DIRECTION ( 'NONE',  ( 0.8660254037844361541, 0.5000000000000042188, 0.000000000000000000 ) ) ;
#5802=DIRECTION ( 'NONE',  ( -0.5000000000000044409, 0.8660254037844360431, 0.000000000000000000 ) ) ;
#5814=ORIENTED_EDGE ( 'NONE', *, *, #1738, .F. ) ;
#5816=FACE_OUTER_BOUND ( 'NONE', #3455, .T. ) ;
#5839=ADVANCED_FACE ( 'NONE', ( #4250 ), #5154, .T. ) ;
#5869=LINE ( 'NONE', #5077, #11380 ) ;
#5873=ORIENTED_EDGE ( 'NONE', *, *, #136, .T. ) ;
#5882=FACE_OUTER_BOUND ( 'NONE', #12700, .T. ) ;
#5897=DIRECTION ( 'NONE',  ( 0.000000000000000000, 0.000000000000000000, 1.000000000000000000 ) ) ;
#5903=DIRECTION ( 'NONE',  ( 0.5000000000000036637, -0.8660254037844365982, 0.000000000000000000 ) ) ;
#5908=CARTESIAN_POINT ( 'NONE',  ( -56.05384757729341061, 33.16506350946112036, 0.000000000000000000 ) ) ;
#5910=LINE ( 'NONE', #1003, #1551 ) ;
#5923=DIRECTION ( 'NONE',  ( 0.000000000000000000, -1.000000000000000000, 0.000000000000000000 ) ) ;
#5924=CARTESIAN_POINT ( 'NONE',  ( -3.666666666666651420, 64.83346624110779999, 2.999999999999900968 ) ) ;
#5925=DIRECTION ( 'NONE',  ( 0.000000000000000000, -1.000000000000000000, 0.000000000000000000 ) ) ;
#5976=DIRECTION ( 'NONE',  ( 0.000000000000000000, 0.000000000000000000, 1.000000000000000000 ) ) ;
#5986=AXIS2_PLACEMENT_3D ( 'NONE', #7038, #8023, #6050 ) ;
#5988=LINE ( 'NONE', #4827, #9365 ) ;
#5994=LINE ( 'NONE', #1948, #8677 ) ;
#6001=CARTESIAN_POINT ( 'NONE',  ( 6.500000000000000000, 68.39379290111055809, -1.000000000000000222 ) ) ;
#6005=ORIENTED_EDGE ( 'NONE', *, *, #4184, .F. ) ;
#6021=CARTESIAN_POINT ( 'NONE',  ( -60.00000000000000000, 30.00000000000000000, -3.000000000000000000 ) ) ;
#6050=DIRECTION ( 'NONE',  ( 0.5000000000000038858, -0.8660254037844362651, 0.000000000000000000 ) ) ;
#6051=ORIENTED_EDGE ( 'NONE', *, *, #1799, .T. ) ;
#6102=DIRECTION ( 'NONE',  ( -0.5000000000000045519, 0.8660254037844360431, 0.000000000000000000 ) ) ;
#6113=ORIENTED_EDGE ( 'NONE', *, *, #9318, .F. ) ;
#6116=CARTESIAN_POINT ( 'NONE',  ( -56.80384757729341771, 34.46410161513777837, 0.000000000000000000 ) ) ;
#6133=ORIENTED_EDGE ( 'NONE', *, *, #7308, .T. ) ;
#6169=CARTESIAN_POINT ( 'NONE',  ( -65.00000000000004263, 38.66025403784436065, 3.000000000000000000 ) ) ;
#6180=DIRECTION ( 'NONE',  ( 0.000000000000000000, -1.000000000000000000, 0.000000000000000000 ) ) ;
#6217=CARTESIAN_POINT ( 'NONE',  ( -60.00000000000000000, 30.00000000000000000, 0.9999999999999926725 ) ) ;
#6231=ORIENTED_EDGE ( 'NONE', *, *, #1962, .F. ) ;
#6254=EDGE_CURVE ( 'NONE', #7039, #9204, #7093, .T. ) ;
#6255=CARTESIAN_POINT ( 'NONE',  ( 8.999999999999987566, 72.14656965084313356, 3.000000000000000000 ) ) ;
#6263=ORIENTED_EDGE ( 'NONE', *, *, #3837, .F. ) ;
#6269=ORIENTED_EDGE ( 'NONE', *, *, #7598, .F. ) ;
#6270=VECTOR ( 'NONE', #7162, 1000.000000000000000 ) ;
#6285=DIRECTION ( 'NONE',  ( 0.000000000000000000, 0.000000000000000000, -1.000000000000000000 ) ) ;
#6296=LINE ( 'NONE', #5318, #11537 ) ;
#6312=ORIENTED_EDGE ( 'NONE', *, *, #10407, .F. ) ;
#6316=DIRECTION ( 'NONE',  ( -0.5000000000000036637, 0.8660254037844365982, 0.000000000000000000 ) ) ;
#6317=LINE ( 'NONE', #6255, #12410 ) ;
#6318=ORIENTED_EDGE ( 'NONE', *, *, #11009, .F. ) ;
#6398=DIRECTION ( 'NONE',  ( -0.000000000000000000, 0.000000000000000000, 1.000000000000000000 ) ) ;
#6408=VERTEX_POINT ( 'NONE', #7480 ) ;
#6461=PRODUCT_DEFINITION_SHAPE ( 'NONE', 'NONE',  #5290 ) ;
#6469=ORIENTED_EDGE ( 'NONE', *, *, #3442, .F. ) ;
#6485=VECTOR ( 'NONE', #685, 1000.000000000000114 ) ;
#6486=CARTESIAN_POINT ( 'NONE',  ( 8.499999999999998224, 71.85789451624832225, 1.000000000000000000 ) ) ;
#6511=ORIENTED_EDGE ( 'NONE', *, *, #10803, .T. ) ;
#6514=EDGE_LOOP ( 'NONE', ( #7462, #11770, #2046, #9962 ) ) ;
#6517=VERTEX_POINT ( 'NONE', #12300 ) ;
#6518=ADVANCED_FACE ( 'NONE', ( #11312 ), #377, .F. ) ;
#6522=EDGE_CURVE ( 'NONE', #5066, #10861, #8249, .T. ) ;
#6568=LINE ( 'NONE', #477, #3717 ) ;
#6575=VECTOR ( 'NONE', #1543, 1000.000000000000000 ) ;
#6579=AXIS2_PLACEMENT_3D ( 'NONE', #4720, #6735, #4908 ) ;
#6590=EDGE_CURVE ( 'NONE', #4892, #8770, #803, .T. ) ;
#6606=UNCERTAINTY_MEASURE_WITH_UNIT (LENGTH_MEASURE( 1.000000000000000082E-05 ), #8219, 'distance_accuracy_value', 'NONE');
#6616=CARTESIAN_POINT ( 'NONE',  ( -61.13397459621560159, 31.96410161513775350, 0.000000000000000000 ) ) ;
#6628=DIRECTION ( 'NONE',  ( -0.000000000000000000, -0.000000000000000000, -1.000000000000000000 ) ) ;
#6656=PLANE ( 'NONE',  #9510 ) ;
#6661=ORIENTED_EDGE ( 'NONE', *, *, #10289, .F. ) ;
#6671=EDGE_CURVE ( 'NONE', #1989, #443, #11335, .T. ) ;
#6673=ORIENTED_EDGE ( 'NONE', *, *, #8569, .T. ) ;
#6675=EDGE_LOOP ( 'NONE', ( #2205, #1885, #6469, #5048 ) ) ;
#6735=DIRECTION ( 'NONE',  ( 1.000000000000000000, 0.000000000000000000, -0.000000000000000000 ) ) ;
#6739=ORIENTED_EDGE ( 'NONE', *, *, #2003, .T. ) ;
#6753=DIRECTION ( 'NONE',  ( -0.000000000000000000, -0.000000000000000000, -1.000000000000000000 ) ) ;
#6780=ORIENTED_EDGE ( 'NONE', *, *, #10388, .T. ) ;
#6784=CARTESIAN_POINT ( 'NONE',  ( -28.99038105676692112, 50.21281292110204930, -1.000000000000000000 ) ) ;
#6794=AXIS2_PLACEMENT_3D ( 'NONE', #12808, #12878, #6980 ) ;
#6820=ORIENTED_EDGE ( 'NONE', *, *, #500, .F. ) ;
#6821=CONICAL_SURFACE ( 'NONE', #3498, 1.500000000000003331, 1.029744259999999967 ) ;
#6840=VECTOR ( 'NONE', #10883, 1000.000000000000114 ) ;
#6847=LINE ( 'NONE', #5924, #3002 ) ;
#6855=DIRECTION ( 'NONE',  ( 0.8660254037844361541, 0.5000000000000042188, 0.000000000000000000 ) ) ;
#6860=ADVANCED_FACE ( 'NONE', ( #3886 ), #6944, .T. ) ;
#6871=ORIENTED_EDGE ( 'NONE', *, *, #2856, .T. ) ;
#6893=ORIENTED_EDGE ( 'NONE', *, *, #3837, .T. ) ;
#6909=AXIS2_PLACEMENT_3D ( 'NONE', #6616, #2642, #11460 ) ;
#6941=VECTOR ( 'NONE', #11053, 1000.000000000000000 ) ;
#6944=PLANE ( 'NONE',  #384 ) ;
#6980=DIRECTION ( 'NONE',  ( 0.5000000000000049960, -0.8660254037844357100, 0.000000000000000000 ) ) ;
#6994=AXIS2_PLACEMENT_3D ( 'NONE', #9248, #10232, #3377 ) ;
#7002=VECTOR ( 'NONE', #486, 1000.000000000000000 ) ;
#7006=AXIS2_PLACEMENT_3D ( 'NONE', #570, #8573, #6398 ) ;
#7017=PLANE ( 'NONE',  #4488 ) ;
#7029=CARTESIAN_POINT ( 'NONE',  ( -61.00000000000000711, 31.73205080756887142, 3.000000000000000000 ) ) ;
#7038=CARTESIAN_POINT ( 'NONE',  ( -56.80384757729341771, 34.46410161513777837, 0.000000000000000000 ) ) ;
#7039=VERTEX_POINT ( 'NONE', #6021 ) ;
#7045=VERTEX_POINT ( 'NONE', #4982 ) ;
#7052=DIRECTION ( 'NONE',  ( 4.336808689942017243E-16, 2.503857664561960972E-16, -1.000000000000000000 ) ) ;
#7066=VECTOR ( 'NONE', #11825, 1000.000000000000000 ) ;
#7093=LINE ( 'NONE', #4346, #10424 ) ;
#7097=EDGE_CURVE ( 'NONE', #3601, #9525, #695, .T. ) ;
#7157=DIRECTION ( 'NONE',  ( -1.000000000000000000, 0.000000000000000000, -0.000000000000000000 ) ) ;
#7159=DIRECTION ( 'NONE',  ( 0.8660254037844361541, 0.5000000000000042188, 0.000000000000000000 ) ) ;
#7162=DIRECTION ( 'NONE',  ( 0.000000000000000000, -1.000000000000000000, 0.000000000000000000 ) ) ;
#7164=EDGE_LOOP ( 'NONE', ( #568, #5214, #4868, #4527 ) ) ;
#7165=COLOUR_RGB ( '',0.8941176470588234615, 0.8941176470588234615, 0.8941176470588234615 ) ;
#7185=CARTESIAN_POINT ( 'NONE',  ( -9.666666666666658969, 79.07477288111861924, 0.9999999999999997780 ) ) ;
#7195=ORIENTED_EDGE ( 'NONE', *, *, #3696, .F. ) ;
#7213=DIRECTION ( 'NONE',  ( 0.000000000000000000, -1.000000000000000000, 0.000000000000000000 ) ) ;
#7224=EDGE_CURVE ( 'NONE', #10861, #8585, #5615, .T. ) ;
#7235=DIRECTION ( 'NONE',  ( 0.8660254037844361541, 0.5000000000000042188, 0.000000000000000000 ) ) ;
#7237=DIRECTION ( 'NONE',  ( -0.8660254037844361541, -0.5000000000000042188, 0.000000000000000000 ) ) ;
#7264=ORIENTED_EDGE ( 'NONE', *, *, #9805, .T. ) ;
#7308=EDGE_CURVE ( 'NONE', #5354, #10861, #5988, .T. ) ;
#7317=ORIENTED_EDGE ( 'NONE', *, *, #136, .F. ) ;
#7318=AXIS2_PLACEMENT_3D ( 'NONE', #11556, #12737, #2602 ) ;
#7337=AXIS2_PLACEMENT_3D ( 'NONE', #5641, #7669, #12516 ) ;
#7362=EDGE_CURVE ( 'NONE', #3514, #3599, #7831, .T. ) ;
#7383=PLANE ( 'NONE',  #7006 ) ;
#7400=ORIENTED_EDGE ( 'NONE', *, *, #7737, .F. ) ;
#7410=LINE ( 'NONE', #12584, #1182 ) ;
#7429=CARTESIAN_POINT ( 'NONE',  ( -31.49999999999998579, 48.76388374866304076, 3.000000000000000000 ) ) ;
#7438=EDGE_LOOP ( 'NONE', ( #7317, #9649, #164, #5664 ) ) ;
#7441=ORIENTED_EDGE ( 'NONE', *, *, #9262, .F. ) ;
#7462=ORIENTED_EDGE ( 'NONE', *, *, #11466, .F. ) ;
#7468=ADVANCED_FACE ( 'NONE', ( #12146 ), #1423, .F. ) ;
#7477=CARTESIAN_POINT ( 'NONE',  ( -3.666666666666661634, 79.07477288111861924, -1.000000000000000666 ) ) ;
#7480=CARTESIAN_POINT ( 'NONE',  ( -31.49999999999998579, 48.76388374866304076, -1.000000000000000000 ) ) ;
#7491=ORIENTED_EDGE ( 'NONE', *, *, #2772, .F. ) ;
#7496=SHAPE_REPRESENTATION_RELATIONSHIP ( 'NONE' , 'NONE' ,  #9937, #10604 ) ;
#7503=LINE ( 'NONE', #8678, #11599 ) ;
#7507=ORIENTED_EDGE ( 'NONE', *, *, #5500, .F. ) ;
#7537=VECTOR ( 'NONE', #6180, 1000.000000000000000 ) ;
#7552=VECTOR ( 'NONE', #12898, 1000.000000000000000 ) ;
#7553=CARTESIAN_POINT ( 'NONE',  ( -23.49999999999999289, 51.07328482542158810, 3.000000000000000000 ) ) ;
#7562=LINE ( 'NONE', #8550, #12413 ) ;
#7568=ORIENTED_EDGE ( 'NONE', *, *, #10389, .F. ) ;
#7569=DIRECTION ( 'NONE',  ( -0.000000000000000000, -0.000000000000000000, -1.000000000000000000 ) ) ;
#7579=ORIENTED_EDGE ( 'NONE', *, *, #3992, .F. ) ;
#7598=EDGE_CURVE ( 'NONE', #1482, #2334, #7562, .T. ) ;
#7601=VERTEX_POINT ( 'NONE', #2594 ) ;
#7641=VECTOR ( 'NONE', #8866, 1000.000000000000000 ) ;
#7645=CARTESIAN_POINT ( 'NONE',  ( -56.05384757729341061, 33.16506350946112036, 0.000000000000000000 ) ) ;
#7669=DIRECTION ( 'NONE',  ( -1.000000000000000000, 0.000000000000000000, 1.301042606982605321E-15 ) ) ;
#7689=( NAMED_UNIT ( * ) PLANE_ANGLE_UNIT ( ) SI_UNIT ( $, .RADIAN. ) );
#7699=CARTESIAN_POINT ( 'NONE',  ( -53.33333333333332149, 79.07477288111861924, -1.000000000000000000 ) ) ;
#7701=LINE ( 'NONE', #2479, #10598 ) ;
#7737=EDGE_CURVE ( 'NONE', #12915, #1292, #11934, .T. ) ;
#7739=VECTOR ( 'NONE', #5794, 1000.000000000000114 ) ;
#7742=CARTESIAN_POINT ( 'NONE',  ( -65.00000000000004263, 38.66025403784436065, -3.000000000000000000 ) ) ;
#7745=DIRECTION ( 'NONE',  ( 8.673617379884034486E-16, 5.007715329123921945E-16, -1.000000000000000000 ) ) ;
#7767=LINE ( 'NONE', #3980, #690 ) ;
#7778=DIRECTION ( 'NONE',  ( -0.8660254037844361541, -0.5000000000000042188, 0.000000000000000000 ) ) ;
#7780=EDGE_CURVE ( 'NONE', #4305, #8971, #5910, .T. ) ;
#7828=CARTESIAN_POINT ( 'NONE',  ( 9.999999999999994671, 70.41451884327426569, 3.000000000000000000 ) ) ;
#7829=ADVANCED_FACE ( 'NONE', ( #5790 ), #3773, .T. ) ;
#7831=LINE ( 'NONE', #1079, #7066 ) ;
#7852=ORIENTED_EDGE ( 'NONE', *, *, #6522, .F. ) ;
#7860=CARTESIAN_POINT ( 'NONE',  ( -54.07179676972453564, 35.73205080756889629, -1.000000000000000000 ) ) ;
#7864=VECTOR ( 'NONE', #1602, 1000.000000000000000 ) ;
#7866=DIRECTION ( 'NONE',  ( -0.8660254037844361541, -0.5000000000000042188, 0.000000000000000000 ) ) ;
#7895=CARTESIAN_POINT ( 'NONE',  ( 6.499999999999999112, 79.07477288111861924, 0.9999999999999997780 ) ) ;
#7900=LINE ( 'NONE', #6784, #11571 ) ;
#7903=ADVANCED_FACE ( 'NONE', ( #269 ), #8340, .T. ) ;
#7910=ADVANCED_FACE ( 'NONE', ( #12264 ), #78, .T. ) ;
#7945=ORIENTED_EDGE ( 'NONE', *, *, #9262, .T. ) ;
#7972=VERTEX_POINT ( 'NONE', #8470 ) ;
#8023=DIRECTION ( 'NONE',  ( -0.8660254037844360431, -0.5000000000000047740, -0.000000000000000000 ) ) ;
#8064=EDGE_CURVE ( 'NONE', #9137, #3599, #1525, .T. ) ;
#8117=VERTEX_POINT ( 'NONE', #11727 ) ;
#8119=DIRECTION ( 'NONE',  ( 0.5000000000000049960, -0.8660254037844357100, 0.000000000000000000 ) ) ;
#8129=AXIS2_PLACEMENT_3D ( 'NONE', #180, #3219, #4132 ) ;
#8153=VERTEX_POINT ( 'NONE', #10931 ) ;
#8206=DIRECTION ( 'NONE',  ( -0.8660254037844362651, -0.5000000000000042188, 0.000000000000000000 ) ) ;
#8219=( LENGTH_UNIT ( ) NAMED_UNIT ( * ) SI_UNIT ( .MILLI., .METRE. ) );
#8237=DIRECTION ( 'NONE',  ( -0.8660254037844361541, -0.5000000000000042188, 0.000000000000000000 ) ) ;
#8240=ORIENTED_EDGE ( 'NONE', *, *, #11663, .F. ) ;
#8249=LINE ( 'NONE', #11114, #11256 ) ;
#8276=LINE ( 'NONE', #10233, #3337 ) ;
#8279=DIRECTION ( 'NONE',  ( -0.5000000000000043299, 0.8660254037844362651, 0.000000000000000000 ) ) ;
#8282=CARTESIAN_POINT ( 'NONE',  ( 8.999999999999989342, 72.14656965084313356, 1.000000000000000000 ) ) ;
#8285=ORIENTED_EDGE ( 'NONE', *, *, #6671, .T. ) ;
#8291=CARTESIAN_POINT ( 'NONE',  ( 4.999999999999962697, 79.07477288111861924, 3.000000000000000000 ) ) ;
#8309=FACE_OUTER_BOUND ( 'NONE', #7164, .T. ) ;
#8310=ORIENTED_EDGE ( 'NONE', *, *, #8901, .T. ) ;
#8325=AXIS2_PLACEMENT_3D ( 'NONE', #6116, #1144, #9263 ) ;
#8340=PLANE ( 'NONE',  #6994 ) ;
#8359=DIRECTION ( 'NONE',  ( 0.8660254037844361541, 0.5000000000000042188, 0.000000000000000000 ) ) ;
#8361=ADVANCED_FACE ( 'NONE', ( #5882 ), #902, .T. ) ;
#8372=VECTOR ( 'NONE', #7569, 1000.000000000000000 ) ;
#8392=CARTESIAN_POINT ( 'NONE',  ( -53.33333333333332149, 36.15840287135605990, -1.000000000000000000 ) ) ;
#8410=FACE_OUTER_BOUND ( 'NONE', #10191, .T. ) ;
#8442=LINE ( 'NONE', #12693, #11816 ) ;
#8459=PRODUCT ( 'sorter block', 'sorter block', '', ( #2619 ) ) ;
#8470=CARTESIAN_POINT ( 'NONE',  ( -23.49999999999998934, 51.07328482542158810, -1.000000000000000000 ) ) ;
#8504=DIRECTION ( 'NONE',  ( 0.000000000000000000, 0.000000000000000000, 1.000000000000000000 ) ) ;
#8542=EDGE_CURVE ( 'NONE', #4807, #3419, #8957, .T. ) ;
#8543=CARTESIAN_POINT ( 'NONE',  ( -60.00000000000000000, 30.00000000000000000, 3.000000000000000000 ) ) ;
#8550=CARTESIAN_POINT ( 'NONE',  ( 4.999999999999962697, 79.07477288111861924, -3.000000000000000000 ) ) ;
#8569=EDGE_CURVE ( 'NONE', #3419, #9344, #5159, .T. ) ;
#8573=DIRECTION ( 'NONE',  ( -1.000000000000000000, 0.000000000000000000, -0.000000000000000000 ) ) ;
#8581=CIRCLE ( 'NONE', #7318, 1.500000000000000222 ) ;
#8585=VERTEX_POINT ( 'NONE', #4512 ) ;
#8610=EDGE_LOOP ( 'NONE', ( #7579, #12098, #12887, #160 ) ) ;
#8615=CARTESIAN_POINT ( 'NONE',  ( 6.500000000000005329, 68.39379290111055809, 3.000000000000038636 ) ) ;
#8627=DIRECTION ( 'NONE',  ( 0.8660254037844361541, 0.5000000000000042188, -9.389466242107225456E-17 ) ) ;
#8654=CLOSED_SHELL ( 'NONE', ( #3977, #1466, #11868, #8752, #1092, #2040, #5839, #4796, #6860, #7829, #2998, #5194, #2498, #12616, #7910, #7903, #11350, #8361, #8657, #3766, #2766, #8687, #12922, #2168, #6518, #7468 ) ) ;
#8657=ADVANCED_FACE ( 'NONE', ( #8309 ), #2357, .T. ) ;
#8663=VECTOR ( 'NONE', #5976, 1000.000000000000000 ) ;
#8677=VECTOR ( 'NONE', #12020, 1000.000000000000000 ) ;
#8678=CARTESIAN_POINT ( 'NONE',  ( -60.00000000000000000, 30.00000000000000000, -0.9999999999999991118 ) ) ;
#8687=ADVANCED_FACE ( 'NONE', ( #5416 ), #7383, .T. ) ;
#8694=CARTESIAN_POINT ( 'NONE',  ( 0.000000000000000000, 0.000000000000000000, 1.000000000000000000 ) ) ;
#8700=EDGE_LOOP ( 'NONE', ( #7568, #11112, #6673, #4248 ) ) ;
#8707=VECTOR ( 'NONE', #728, 1000.000000000000000 ) ;
#8750=DIRECTION ( 'NONE',  ( -0.8660254037844361541, -0.5000000000000042188, 9.389466242107221759E-17 ) ) ;
#8752=ADVANCED_FACE ( 'NONE', ( #11761 ), #6656, .T. ) ;
#8770=VERTEX_POINT ( 'NONE', #7645 ) ;
#8789=CARTESIAN_POINT ( 'NONE',  ( -23.49999999999999289, 51.07328482542158810, 1.000000000000000000 ) ) ;
#8814=LINE ( 'NONE', #10899, #12820 ) ;
#8832=CARTESIAN_POINT ( 'NONE',  ( 4.999999999999962697, 79.07477288111861924, 1.000000000000000000 ) ) ;
#8836=STYLED_ITEM ( 'NONE', ( #11348 ), #10604 ) ;
#8863=DIRECTION ( 'NONE',  ( -0.5000000000000043299, 0.8660254037844362651, 0.000000000000000000 ) ) ;
#8866=DIRECTION ( 'NONE',  ( 0.8660254037844361541, 0.5000000000000042188, 0.000000000000000000 ) ) ;
#8867=CARTESIAN_POINT ( 'NONE',  ( 4.999999999999962697, 79.07477288111861924, 3.000000000000000000 ) ) ;
#8892=CARTESIAN_POINT ( 'NONE',  ( 8.499999999999998224, 71.85789451624832225, -1.000000000000000222 ) ) ;
#8901=EDGE_CURVE ( 'NONE', #10113, #1516, #8276, .T. ) ;
#8911=EDGE_CURVE ( 'NONE', #12578, #12915, #11142, .T. ) ;
#8925=CARTESIAN_POINT ( 'NONE',  ( 8.499999999999992895, 69.54849343948981755, 3.000000000000000000 ) ) ;
#8930=CARTESIAN_POINT ( 'NONE',  ( -53.33333333333332149, 79.07477288111861924, -1.000000000000000000 ) ) ;
#8938=EDGE_CURVE ( 'NONE', #2627, #3833, #1328, .T. ) ;
#8954=ORIENTED_EDGE ( 'NONE', *, *, #7097, .T. ) ;
#8957=LINE ( 'NONE', #11108, #2628 ) ;
#8971=VERTEX_POINT ( 'NONE', #10900 ) ;
#8997=CARTESIAN_POINT ( 'NONE',  ( 0.000000000000000000, 0.000000000000000000, 0.000000000000000000 ) ) ;
#9017=ORIENTED_EDGE ( 'NONE', *, *, #9162, .F. ) ;
#9038=ORIENTED_EDGE ( 'NONE', *, *, #6590, .T. ) ;
#9053=CARTESIAN_POINT ( 'NONE',  ( -32.99038105676694954, 57.14101615137754209, -1.000000000000000000 ) ) ;
#9102=AXIS2_PLACEMENT_3D ( 'NONE', #8291, #1282, #6316 ) ;
#9124=CARTESIAN_POINT ( 'NONE',  ( -28.99038105676692112, 50.21281292110204930, 1.000000000000000000 ) ) ;
#9137=VERTEX_POINT ( 'NONE', #667 ) ;
#9146=VECTOR ( 'NONE', #12383, 1000.000000000000000 ) ;
#9162=EDGE_CURVE ( 'NONE', #11802, #12915, #9577, .T. ) ;
#9171=ORIENTED_EDGE ( 'NONE', *, *, #3260, .T. ) ;
#9172=VECTOR ( 'NONE', #5127, 1000.000000000000000 ) ;
#9195=SURFACE_SIDE_STYLE ('',( #3123 ) ) ;
#9203=CARTESIAN_POINT ( 'NONE',  ( -3.666666666666658969, 64.83346624110779999, 1.000000000000000000 ) ) ;
#9204=VERTEX_POINT ( 'NONE', #7742 ) ;
#9221=FACE_OUTER_BOUND ( 'NONE', #11438, .T. ) ;
#9248=CARTESIAN_POINT ( 'NONE',  ( -9.666666666666657193, 79.07477288111861924, -1.000000000000000000 ) ) ;
#9262=EDGE_CURVE ( 'NONE', #443, #12930, #5046, .T. ) ;
#9263=DIRECTION ( 'NONE',  ( 0.5000000000000038858, -0.8660254037844362651, 0.000000000000000000 ) ) ;
#9268=CARTESIAN_POINT ( 'NONE',  ( -32.99038105676694954, 57.14101615137754209, 1.000000000000000000 ) ) ;
#9279=ORIENTED_EDGE ( 'NONE', *, *, #1473, .T. ) ;
#9301=VECTOR ( 'NONE', #8359, 1000.000000000000000 ) ;
#9302=EDGE_CURVE ( 'NONE', #1989, #9204, #922, .T. ) ;
#9318=EDGE_CURVE ( 'NONE', #2314, #8971, #10873, .T. ) ;
#9344=VERTEX_POINT ( 'NONE', #1383 ) ;
#9348=DIRECTION ( 'NONE',  ( -1.000000000000000000, 0.000000000000000000, 0.000000000000000000 ) ) ;
#9357=EDGE_CURVE ( 'NONE', #3419, #2347, #12314, .T. ) ;
#9365=VECTOR ( 'NONE', #5923, 1000.000000000000000 ) ;
#9382=CARTESIAN_POINT ( 'NONE',  ( -53.07079676972452376, 33.99826794919245998, -1.000000000000000000 ) ) ;
#9404=DIRECTION ( 'NONE',  ( -1.000000000000000000, 0.000000000000000000, -0.000000000000000000 ) ) ;
#9417=ORIENTED_EDGE ( 'NONE', *, *, #8901, .F. ) ;
#9426=EDGE_LOOP ( 'NONE', ( #2435, #9683, #11655, #1161 ) ) ;
#9437=VECTOR ( 'NONE', #7052, 1000.000000000000000 ) ;
#9444=DIRECTION ( 'NONE',  ( 0.8660254037844361541, 0.5000000000000042188, 0.000000000000000000 ) ) ;
#9476=ORIENTED_EDGE ( 'NONE', *, *, #4971, .T. ) ;
#9493=EDGE_LOOP ( 'NONE', ( #724, #9617, #6893, #10266 ) ) ;
#9510=AXIS2_PLACEMENT_3D ( 'NONE', #8694, #10781, #10651 ) ;
#9515=CARTESIAN_POINT ( 'NONE',  ( -9.666666666666657193, 59.05996354921150271, -1.000000000000000222 ) ) ;
#9525=VERTEX_POINT ( 'NONE', #8392 ) ;
#9529=DIRECTION ( 'NONE',  ( -0.000000000000000000, -0.000000000000000000, -1.000000000000000000 ) ) ;
#9577=LINE ( 'NONE', #5713, #4374 ) ;
#9580=CARTESIAN_POINT ( 'NONE',  ( -9.666666666666657193, 61.36936462597000741, 3.000000000000059508 ) ) ;
#9617=ORIENTED_EDGE ( 'NONE', *, *, #1675, .T. ) ;
#9649=ORIENTED_EDGE ( 'NONE', *, *, #3442, .T. ) ;
#9655=LINE ( 'NONE', #8615, #7002 ) ;
#9668=AXIS2_PLACEMENT_3D ( 'NONE', #3207, #5409, #9404 ) ;
#9678=VERTEX_POINT ( 'NONE', #8832 ) ;
#9683=ORIENTED_EDGE ( 'NONE', *, *, #3799, .F. ) ;
#9731=PRODUCT_DEFINITION_CONTEXT ( 'detailed design', #11442, 'design' ) ;
#9749=ORIENTED_EDGE ( 'NONE', *, *, #4858, .F. ) ;
#9756=ORIENTED_EDGE ( 'NONE', *, *, #1293, .T. ) ;
#9771=CARTESIAN_POINT ( 'NONE',  ( -60.00000000000000000, 30.00000000000000000, 3.000000000000000000 ) ) ;
#9805=EDGE_CURVE ( 'NONE', #10254, #8117, #9925, .T. ) ;
#9853=CARTESIAN_POINT ( 'NONE',  ( -53.07079676972452376, 33.99826794919245998, 1.000000000000000000 ) ) ;
#9906=CARTESIAN_POINT ( 'NONE',  ( -31.49999999999998579, 79.07477288111861924, -1.000000000000000000 ) ) ;
#9913=FACE_OUTER_BOUND ( 'NONE', #11095, .T. ) ;
#9925=LINE ( 'NONE', #11831, #11065 ) ;
#9937=SHAPE_REPRESENTATION ( 'sorter block', ( #5704 ), #258 ) ;
#9962=ORIENTED_EDGE ( 'NONE', *, *, #12932, .F. ) ;
#9964=CIRCLE ( 'NONE', #5986, 1.500000000000003331 ) ;
#9990=DIRECTION ( 'NONE',  ( 0.000000000000000000, -1.000000000000000000, 0.000000000000000000 ) ) ;
#9998=ORIENTED_EDGE ( 'NONE', *, *, #4406, .T. ) ;
#10021=EDGE_CURVE ( 'NONE', #9204, #1482, #159, .T. ) ;
#10036=DIRECTION ( 'NONE',  ( 0.000000000000000000, -1.000000000000000000, 0.000000000000000000 ) ) ;
#10056=( GEOMETRIC_REPRESENTATION_CONTEXT ( 3 ) GLOBAL_UNCERTAINTY_ASSIGNED_CONTEXT ( ( #3326 ) ) GLOBAL_UNIT_ASSIGNED_CONTEXT ( ( #11835, #10850, #3928 ) ) REPRESENTATION_CONTEXT ( 'NONE', 'WORKASPACE' ) );
#10063=DIRECTION ( 'NONE',  ( 0.000000000000000000, 0.000000000000000000, 1.000000000000000000 ) ) ;
#10070=ORIENTED_EDGE ( 'NONE', *, *, #4651, .T. ) ;
#10078=ORIENTED_EDGE ( 'NONE', *, *, #10426, .T. ) ;
#10113=VERTEX_POINT ( 'NONE', #9203 ) ;
#10169=DIRECTION ( 'NONE',  ( 0.000000000000000000, -1.000000000000000000, 0.000000000000000000 ) ) ;
#10191=EDGE_LOOP ( 'NONE', ( #10300, #2163, #9038 ) ) ;
#10198=ORIENTED_EDGE ( 'NONE', *, *, #8938, .F. ) ;
#10208=DIRECTION ( 'NONE',  ( -0.8660254037844359321, -0.5000000000000046629, -0.000000000000000000 ) ) ;
#10218=ORIENTED_EDGE ( 'NONE', *, *, #10679, .F. ) ;
#10232=DIRECTION ( 'NONE',  ( 1.000000000000000000, 0.000000000000000000, 8.673617379884034486E-16 ) ) ;
#10233=CARTESIAN_POINT ( 'NONE',  ( -28.99038105676692112, 50.21281292110204930, 1.000000000000000000 ) ) ;
#10239=EDGE_LOOP ( 'NONE', ( #12426, #2537, #240, #5540 ) ) ;
#10253=CARTESIAN_POINT ( 'NONE',  ( 8.500000000000000000, 71.85789451624832225, 3.000000000000000000 ) ) ;
#10254=VERTEX_POINT ( 'NONE', #11554 ) ;
#10266=ORIENTED_EDGE ( 'NONE', *, *, #4858, .T. ) ;
#10279=ORIENTED_EDGE ( 'NONE', *, *, #10389, .T. ) ;
#10289=EDGE_CURVE ( 'NONE', #3204, #4892, #1742, .T. ) ;
#10300=ORIENTED_EDGE ( 'NONE', *, *, #4971, .F. ) ;
#10305=( NAMED_UNIT ( * ) SI_UNIT ( $, .STERADIAN. ) SOLID_ANGLE_UNIT ( ) );
#10326=VECTOR ( 'NONE', #10763, 1000.000000000000000 ) ;
#10329=AXIS2_PLACEMENT_3D ( 'NONE', #7029, #8863, #2918 ) ;
#10341=VECTOR ( 'NONE', #2553, 1000.000000000000114 ) ;
#10367=FACE_BOUND ( 'NONE', #8610, .T. ) ;
#10374=( NAMED_UNIT ( * ) SI_UNIT ( $, .STERADIAN. ) SOLID_ANGLE_UNIT ( ) );
#10388=EDGE_CURVE ( 'NONE', #6517, #5066, #3778, .T. ) ;
#10389=EDGE_CURVE ( 'NONE', #4807, #5354, #1617, .T. ) ;
#10402=DIRECTION ( 'NONE',  ( 8.673617379884034486E-16, 5.007715329123921945E-16, -1.000000000000000000 ) ) ;
#10407=EDGE_CURVE ( 'NONE', #4788, #1482, #10701, .T. ) ;
#10424=VECTOR ( 'NONE', #6102, 1000.000000000000114 ) ;
#10426=EDGE_CURVE ( 'NONE', #12446, #255, #8581, .T. ) ;
#10433=LINE ( 'NONE', #11541, #10796 ) ;
#10440=EDGE_CURVE ( 'NONE', #1516, #8153, #10582, .T. ) ;
#10450=DIRECTION ( 'NONE',  ( 0.8660254037844361541, 0.5000000000000042188, 0.000000000000000000 ) ) ;
#10457=EDGE_LOOP ( 'NONE', ( #7507, #7491, #6113, #3937 ) ) ;
#10476=EDGE_CURVE ( 'NONE', #8117, #11802, #11082, .T. ) ;
#10482=PLANE ( 'NONE',  #7337 ) ;
#10495=LINE ( 'NONE', #1531, #7864 ) ;
#10500=ORIENTED_EDGE ( 'NONE', *, *, #1559, .F. ) ;
#10511=VECTOR ( 'NONE', #5802, 1000.000000000000227 ) ;
#10528=SHAPE_DEFINITION_REPRESENTATION ( #6461, #9937 ) ;
#10540=UNCERTAINTY_MEASURE_WITH_UNIT (LENGTH_MEASURE( 1.000000000000000082E-05 ), #2138, 'distance_accuracy_value', 'NONE');
#10559=VECTOR ( 'NONE', #2538, 1000.000000000000227 ) ;
#10566=LINE ( 'NONE', #8543, #3777 ) ;
#10577=CARTESIAN_POINT ( 'NONE',  ( 9.999999999999994671, 70.41451884327426569, 3.000000000000000000 ) ) ;
#10578=VECTOR ( 'NONE', #3525, 1000.000000000000000 ) ;
#10580=CARTESIAN_POINT ( 'NONE',  ( -43.33333333333332860, 41.93190556325237850, 3.000000000000000000 ) ) ;
#10582=LINE ( 'NONE', #4032, #7537 ) ;
#10596=CARTESIAN_POINT ( 'NONE',  ( 8.499999999999992895, 69.54849343948981755, 1.000000000000000000 ) ) ;
#10598=VECTOR ( 'NONE', #5541, 1000.000000000000114 ) ;
#10604=ADVANCED_BREP_SHAPE_REPRESENTATION ( '', ( #11875, #5704 ), #258 ) ;
#10633=DIRECTION ( 'NONE',  ( 0.5000000000000036637, -0.8660254037844365982, 0.000000000000000000 ) ) ;
#10651=DIRECTION ( 'NONE',  ( -1.000000000000000000, 0.000000000000000000, -0.000000000000000000 ) ) ;
#10679=EDGE_CURVE ( 'NONE', #9678, #3833, #5386, .T. ) ;
#10701=LINE ( 'NONE', #8867, #8372 ) ;
#10704=AXIS2_PLACEMENT_3D ( 'NONE', #7895, #12931, #2869 ) ;
#10721=ORIENTED_EDGE ( 'NONE', *, *, #3629, .F. ) ;
#10742=CARTESIAN_POINT ( 'NONE',  ( -61.00000000000000711, 31.73205080756887142, 3.000000000000000000 ) ) ;
#10763=DIRECTION ( 'NONE',  ( 0.000000000000000000, -1.000000000000000000, 0.000000000000000000 ) ) ;
#10776=EDGE_CURVE ( 'NONE', #4584, #7039, #10566, .T. ) ;
#10781=DIRECTION ( 'NONE',  ( 0.000000000000000000, 0.000000000000000000, -1.000000000000000000 ) ) ;
#10787=ORIENTED_EDGE ( 'NONE', *, *, #388, .T. ) ;
#10796=VECTOR ( 'NONE', #4616, 1000.000000000000000 ) ;
#10803=EDGE_CURVE ( 'NONE', #4584, #12930, #12531, .T. ) ;
#10824=AXIS2_PLACEMENT_3D ( 'NONE', #6169, #202, #8206 ) ;
#10836=LINE ( 'NONE', #9853, #10511 ) ;
#10850=( NAMED_UNIT ( * ) PLANE_ANGLE_UNIT ( ) SI_UNIT ( $, .RADIAN. ) );
#10861=VERTEX_POINT ( 'NONE', #9515 ) ;
#10862=EDGE_CURVE ( 'NONE', #7972, #2347, #3763, .T. ) ;
#10870=EDGE_CURVE ( 'NONE', #9344, #5354, #5717, .T. ) ;
#10873=LINE ( 'NONE', #1917, #1663 ) ;
#10883=DIRECTION ( 'NONE',  ( -0.01745240511413415074, -0.9998476951794869061, 0.000000000000000000 ) ) ;
#10899=CARTESIAN_POINT ( 'NONE',  ( -23.49999999999999289, 79.07477288111861924, -1.000000000000000000 ) ) ;
#10900=CARTESIAN_POINT ( 'NONE',  ( -43.33333333333332860, 39.62250448649387380, 0.9999999999999997780 ) ) ;
#10931=CARTESIAN_POINT ( 'NONE',  ( 6.500000000000002665, 68.39379290111055809, 0.9999999999999997780 ) ) ;
#10968=ORIENTED_EDGE ( 'NONE', *, *, #12211, .F. ) ;
#11007=DIRECTION ( 'NONE',  ( 0.8660254037844361541, 0.5000000000000042188, 0.000000000000000000 ) ) ;
#11009=EDGE_CURVE ( 'NONE', #4788, #3097, #3105, .T. ) ;
#11053=DIRECTION ( 'NONE',  ( 0.000000000000000000, -1.000000000000000000, 0.000000000000000000 ) ) ;
#11065=VECTOR ( 'NONE', #6855, 1000.000000000000114 ) ;
#11080=FACE_BOUND ( 'NONE', #10457, .T. ) ;
#11082=LINE ( 'NONE', #3185, #6270 ) ;
#11095=EDGE_LOOP ( 'NONE', ( #2015, #7195, #484, #1711 ) ) ;
#11108=CARTESIAN_POINT ( 'NONE',  ( -23.49999999999999289, 53.38268590218009280, 3.000000000000000000 ) ) ;
#11112=ORIENTED_EDGE ( 'NONE', *, *, #8542, .T. ) ;
#11114=CARTESIAN_POINT ( 'NONE',  ( -9.666666666666657193, 59.05996354921150271, 3.000000000000058176 ) ) ;
#11142=LINE ( 'NONE', #12134, #9172 ) ;
#11150=EDGE_LOOP ( 'NONE', ( #7852, #2372, #2755, #3267 ) ) ;
#11256=VECTOR ( 'NONE', #10402, 1000.000000000000000 ) ;
#11282=DIRECTION ( 'NONE',  ( 0.000000000000000000, -1.000000000000000000, 0.000000000000000000 ) ) ;
#11289=EDGE_CURVE ( 'NONE', #255, #12446, #12568, .T. ) ;
#11312=FACE_OUTER_BOUND ( 'NONE', #2937, .T. ) ;
#11320=CARTESIAN_POINT ( 'NONE',  ( -53.33333333333332149, 36.15840287135605990, 3.000000000000000000 ) ) ;
#11335=LINE ( 'NONE', #2578, #12734 ) ;
#11346=FACE_OUTER_BOUND ( 'NONE', #4973, .T. ) ;
#11348=PRESENTATION_STYLE_ASSIGNMENT (( #12340 ) ) ;
#11350=ADVANCED_FACE ( 'NONE', ( #4534 ), #10482, .T. ) ;
#11363=ORIENTED_EDGE ( 'NONE', *, *, #1766, .T. ) ;
#11380=VECTOR ( 'NONE', #9990, 1000.000000000000000 ) ;
#11389=ORIENTED_EDGE ( 'NONE', *, *, #7308, .F. ) ;
#11425=CARTESIAN_POINT ( 'NONE',  ( -58.07179676972458537, 42.66025403784442460, -1.000000000000000000 ) ) ;
#11438=EDGE_LOOP ( 'NONE', ( #12101, #3593, #4820, #2633 ) ) ;
#11442=APPLICATION_CONTEXT ( 'automotive_design' ) ;
#11444=ORIENTED_EDGE ( 'NONE', *, *, #10021, .F. ) ;
#11460=DIRECTION ( 'NONE',  ( 0.5000000000000049960, -0.8660254037844357100, 0.000000000000000000 ) ) ;
#11463=CARTESIAN_POINT ( 'NONE',  ( -9.666666666666657193, 61.36936462597000741, -1.000000000000000000 ) ) ;
#11466=EDGE_CURVE ( 'NONE', #9137, #41, #4068, .T. ) ;
#11473=DIRECTION ( 'NONE',  ( -0.5000000000000044409, 0.8660254037844360431, 0.000000000000000000 ) ) ;
#11479=ORIENTED_EDGE ( 'NONE', *, *, #1738, .T. ) ;
#11499=VECTOR ( 'NONE', #671, 1000.000000000000114 ) ;
#11515=CARTESIAN_POINT ( 'NONE',  ( -61.88397459621560870, 33.26313972081441506, 1.836970198721030427E-16 ) ) ;
#11524=ORIENTED_EDGE ( 'NONE', *, *, #5188, .T. ) ;
#11529=STYLED_ITEM('',(#12981),#11875);
#11537=VECTOR ( 'NONE', #1323, 1000.000000000000000 ) ;
#11541=CARTESIAN_POINT ( 'NONE',  ( -3.666666666666651420, 62.52406516434930239, 2.999999999999902300 ) ) ;
#11554=CARTESIAN_POINT ( 'NONE',  ( -3.666666666666661634, 64.83346624110779999, -1.000000000000000666 ) ) ;
#11556=CARTESIAN_POINT ( 'NONE',  ( -61.13397459621560159, 31.96410161513775350, 0.000000000000000000 ) ) ;
#11571=VECTOR ( 'NONE', #1819, 1000.000000000000114 ) ;
#11579=ORIENTED_EDGE ( 'NONE', *, *, #500, .T. ) ;
#11593=ORIENTED_EDGE ( 'NONE', *, *, #11009, .T. ) ;
#11598=CARTESIAN_POINT ( 'NONE',  ( -31.49999999999998579, 79.07477288111861924, 1.000000000000000000 ) ) ;
#11599=VECTOR ( 'NONE', #4627, 1000.000000000000114 ) ;
#11602=EDGE_CURVE ( 'NONE', #1292, #8153, #1177, .T. ) ;
#11611=ORIENTED_EDGE ( 'NONE', *, *, #10440, .F. ) ;
#11655=ORIENTED_EDGE ( 'NONE', *, *, #2856, .F. ) ;
#11663=EDGE_CURVE ( 'NONE', #8770, #255, #1245, .T. ) ;
#11676=DIRECTION ( 'NONE',  ( 0.000000000000000000, 0.000000000000000000, -1.000000000000000000 ) ) ;
#11727=CARTESIAN_POINT ( 'NONE',  ( 6.499999999999999112, 70.70319397786906279, -1.000000000000000000 ) ) ;
#11728=CARTESIAN_POINT ( 'NONE',  ( -65.00000000000004263, 38.66025403784436065, 3.000000000000000000 ) ) ;
#11748=CARTESIAN_POINT ( 'NONE',  ( -60.00000000000000000, 30.00000000000000000, 1.000000000000005551 ) ) ;
#11760=( GEOMETRIC_REPRESENTATION_CONTEXT ( 3 ) GLOBAL_UNCERTAINTY_ASSIGNED_CONTEXT ( ( #10540 ) ) GLOBAL_UNIT_ASSIGNED_CONTEXT ( ( #2138, #7689, #10374 ) ) REPRESENTATION_CONTEXT ( 'NONE', 'WORKASPACE' ) );
#11761=FACE_OUTER_BOUND ( 'NONE', #5759, .T. ) ;
#11770=ORIENTED_EDGE ( 'NONE', *, *, #8064, .T. ) ;
#11802=VERTEX_POINT ( 'NONE', #6001 ) ;
#11805=EDGE_LOOP ( 'NONE', ( #11363, #2617, #3893, #11988 ) ) ;
#11816=VECTOR ( 'NONE', #3478, 1000.000000000000114 ) ;
#11825=DIRECTION ( 'NONE',  ( -0.000000000000000000, -0.000000000000000000, -1.000000000000000000 ) ) ;
#11831=CARTESIAN_POINT ( 'NONE',  ( -28.99038105676692112, 50.21281292110204930, -1.000000000000000000 ) ) ;
#11835=( LENGTH_UNIT ( ) NAMED_UNIT ( * ) SI_UNIT ( .MILLI., .METRE. ) );
#11837=EDGE_CURVE ( 'NONE', #1516, #8117, #11958, .T. ) ;
#11868=ADVANCED_FACE ( 'NONE', ( #5816 ), #5024, .T. ) ;
#11875=MANIFOLD_SOLID_BREP ( 'AdvancedHole1', #8654 ) ;
#11894=VECTOR ( 'NONE', #7213, 1000.000000000000000 ) ;
#11895=EDGE_LOOP ( 'NONE', ( #1406, #11389, #878, #576 ) ) ;
#11908=EDGE_LOOP ( 'NONE', ( #11524, #5167, #1337, #896 ) ) ;
#11934=LINE ( 'NONE', #8925, #8663 ) ;
#11944=AXIS2_PLACEMENT_3D ( 'NONE', #3074, #1829, #7778 ) ;
#11958=LINE ( 'NONE', #3800, #9437 ) ;
#11960=PLANE ( 'NONE',  #9668 ) ;
#11970=ORIENTED_EDGE ( 'NONE', *, *, #11602, .F. ) ;
#11985=VERTEX_POINT ( 'NONE', #2089 ) ;
#11988=ORIENTED_EDGE ( 'NONE', *, *, #10440, .T. ) ;
#12011=FACE_OUTER_BOUND ( 'NONE', #11805, .T. ) ;
#12013=PLANE ( 'NONE',  #9102 ) ;
#12020=DIRECTION ( 'NONE',  ( -0.000000000000000000, -0.000000000000000000, -1.000000000000000000 ) ) ;
#12044=LINE ( 'NONE', #7185, #6941 ) ;
#12047=EDGE_CURVE ( 'NONE', #3601, #3649, #6296, .T. ) ;
#12073=LINE ( 'NONE', #5200, #4528 ) ;
#12080=CARTESIAN_POINT ( 'NONE',  ( -60.38397459621558738, 30.66506350946110260, 0.000000000000000000 ) ) ;
#12085=DIRECTION ( 'NONE',  ( 0.8660254037844362651, 0.5000000000000042188, 0.000000000000000000 ) ) ;
#12093=DIRECTION ( 'NONE',  ( -0.5000000000000043299, 0.8660254037844362651, 0.000000000000000000 ) ) ;
#12098=ORIENTED_EDGE ( 'NONE', *, *, #4074, .F. ) ;
#12101=ORIENTED_EDGE ( 'NONE', *, *, #9318, .T. ) ;
#12134=CARTESIAN_POINT ( 'NONE',  ( 8.499999999999998224, 79.07477288111861924, -1.000000000000000222 ) ) ;
#12142=PLANE ( 'NONE',  #3304 ) ;
#12146=FACE_OUTER_BOUND ( 'NONE', #2412, .T. ) ;
#12190=EDGE_LOOP ( 'NONE', ( #7400, #9017, #2180, #11970 ) ) ;
#12206=DIRECTION ( 'NONE',  ( -0.5000000000000043299, 0.8660254037844362651, 0.000000000000000000 ) ) ;
#12211=EDGE_CURVE ( 'NONE', #9344, #5066, #12044, .T. ) ;
#12219=AXIS2_PLACEMENT_3D ( 'NONE', #4095, #4157, #7157 ) ;
#12264=FACE_OUTER_BOUND ( 'NONE', #10239, .T. ) ;
#12300=CARTESIAN_POINT ( 'NONE',  ( -3.666666666666659413, 62.52406516434930239, 0.9999999999999991118 ) ) ;
#12314=LINE ( 'NONE', #2181, #11894 ) ;
#12331=CARTESIAN_POINT ( 'NONE',  ( -60.00000000000000000, 30.00000000000000000, 3.000000000000000000 ) ) ;
#12340=SURFACE_STYLE_USAGE ( .BOTH. , #9195 ) ;
#12351=CARTESIAN_POINT ( 'NONE',  ( -23.49999999999999289, 53.38268590218009280, 1.000000000000000000 ) ) ;
#12365=APPLICATION_CONTEXT ( 'automotive_design' ) ;
#12383=DIRECTION ( 'NONE',  ( 0.000000000000000000, -1.000000000000000000, 0.000000000000000000 ) ) ;
#12388=CARTESIAN_POINT ( 'NONE',  ( -28.99038105676692112, 50.21281292110204930, 1.000000000000000000 ) ) ;
#12393=CARTESIAN_POINT ( 'NONE',  ( -56.80384757729341771, 34.46410161513777837, 0.000000000000000000 ) ) ;
#12410=VECTOR ( 'NONE', #4175, 1000.000000000000000 ) ;
#12413=VECTOR ( 'NONE', #10633, 1000.000000000000000 ) ;
#12426=ORIENTED_EDGE ( 'NONE', *, *, #5188, .F. ) ;
#12446=VERTEX_POINT ( 'NONE', #11515 ) ;
#12448=ORIENTED_EDGE ( 'NONE', *, *, #5266, .T. ) ;
#12453=LINE ( 'NONE', #11598, #9146 ) ;
#12462=VECTOR ( 'NONE', #1156, 1000.000000000000000 ) ;
#12495=LINE ( 'NONE', #3538, #10341 ) ;
#12516=DIRECTION ( 'NONE',  ( 1.301042606982605321E-15, 0.000000000000000000, 1.000000000000000000 ) ) ;
#12528=PLANE ( 'NONE',  #4098 ) ;
#12531=LINE ( 'NONE', #9771, #11499 ) ;
#12568=CIRCLE ( 'NONE', #6909, 1.500000000000000222 ) ;
#12578=VERTEX_POINT ( 'NONE', #8892 ) ;
#12584=CARTESIAN_POINT ( 'NONE',  ( -60.00000000000000000, 30.00000000000000000, 1.000000000000000000 ) ) ;
#12596=EDGE_LOOP ( 'NONE', ( #5093, #5244, #2216, #6051, #3639, #4966, #11579, #9998, #4773, #10279, #6133, #315, #6005, #7264, #3196, #2255, #2867, #5873, #6318, #6231 ) ) ;
#12616=ADVANCED_FACE ( 'NONE', ( #1031 ), #11960, .F. ) ;
#12677=ORIENTED_EDGE ( 'NONE', *, *, #10679, .T. ) ;
#12680=AXIS2_PLACEMENT_3D ( 'NONE', #8930, #1809, #943 ) ;
#12693=CARTESIAN_POINT ( 'NONE',  ( -28.99038105676692112, 50.21281292110204930, 1.000000000000000000 ) ) ;
#12700=EDGE_LOOP ( 'NONE', ( #5670, #6820, #9749, #12448 ) ) ;
#12716=AXIS2_PLACEMENT_3D ( 'NONE', #2229, #12093, #8237 ) ;
#12718=CARTESIAN_POINT ( 'NONE',  ( 4.999999999999962697, 79.07477288111861924, 3.000000000000000000 ) ) ;
#12724=ORIENTED_EDGE ( 'NONE', *, *, #11466, .T. ) ;
#12734=VECTOR ( 'NONE', #5515, 1000.000000000000114 ) ;
#12737=DIRECTION ( 'NONE',  ( -0.8660254037844360431, -0.5000000000000047740, -0.000000000000000000 ) ) ;
#12808=CARTESIAN_POINT ( 'NONE',  ( -61.13397459621560159, 31.96410161513775350, 0.000000000000000000 ) ) ;
#12820=VECTOR ( 'NONE', #5925, 1000.000000000000000 ) ;
#12866=CARTESIAN_POINT ( 'NONE',  ( -60.00000000000000000, 30.00000000000000000, 3.000000000000000000 ) ) ;
#12875=CARTESIAN_POINT ( 'NONE',  ( -54.07179676972453564, 35.73205080756890339, 1.000000000000000000 ) ) ;
#12878=DIRECTION ( 'NONE',  ( -0.8660254037844360431, -0.5000000000000047740, -0.000000000000000000 ) ) ;
#12887=ORIENTED_EDGE ( 'NONE', *, *, #10862, .F. ) ;
#12898=DIRECTION ( 'NONE',  ( 0.000000000000000000, 0.000000000000000000, 1.000000000000000000 ) ) ;
#12912=ORIENTED_EDGE ( 'NONE', *, *, #3799, .T. ) ;
#12915=VERTEX_POINT ( 'NONE', #4949 ) ;
#12922=ADVANCED_FACE ( 'NONE', ( #12011 ), #820, .T. ) ;
#12930=VERTEX_POINT ( 'NONE', #7828 ) ;
#12931=DIRECTION ( 'NONE',  ( 1.000000000000000000, 0.000000000000000000, 4.336808689942017243E-16 ) ) ;
#12932=EDGE_CURVE ( 'NONE', #41, #3514, #10836, .T. ) ;
#12975=COLOUR_RGB('Dark Blue',0.08,0.2,0.34);
#12976=FILL_AREA_STYLE_COLOUR('',#12975);
#12977=FILL_AREA_STYLE('',(#12976));
#12978=SURFACE_STYLE_FILL_AREA(#12977);
#12979=SURFACE_SIDE_STYLE('',(#12978));
#12980=SURFACE_STYLE_USAGE(.BOTH.,#12979);
#12981=PRESENTATION_STYLE_ASSIGNMENT((#12980));
ENDSEC;
END-ISO-10303-21;
